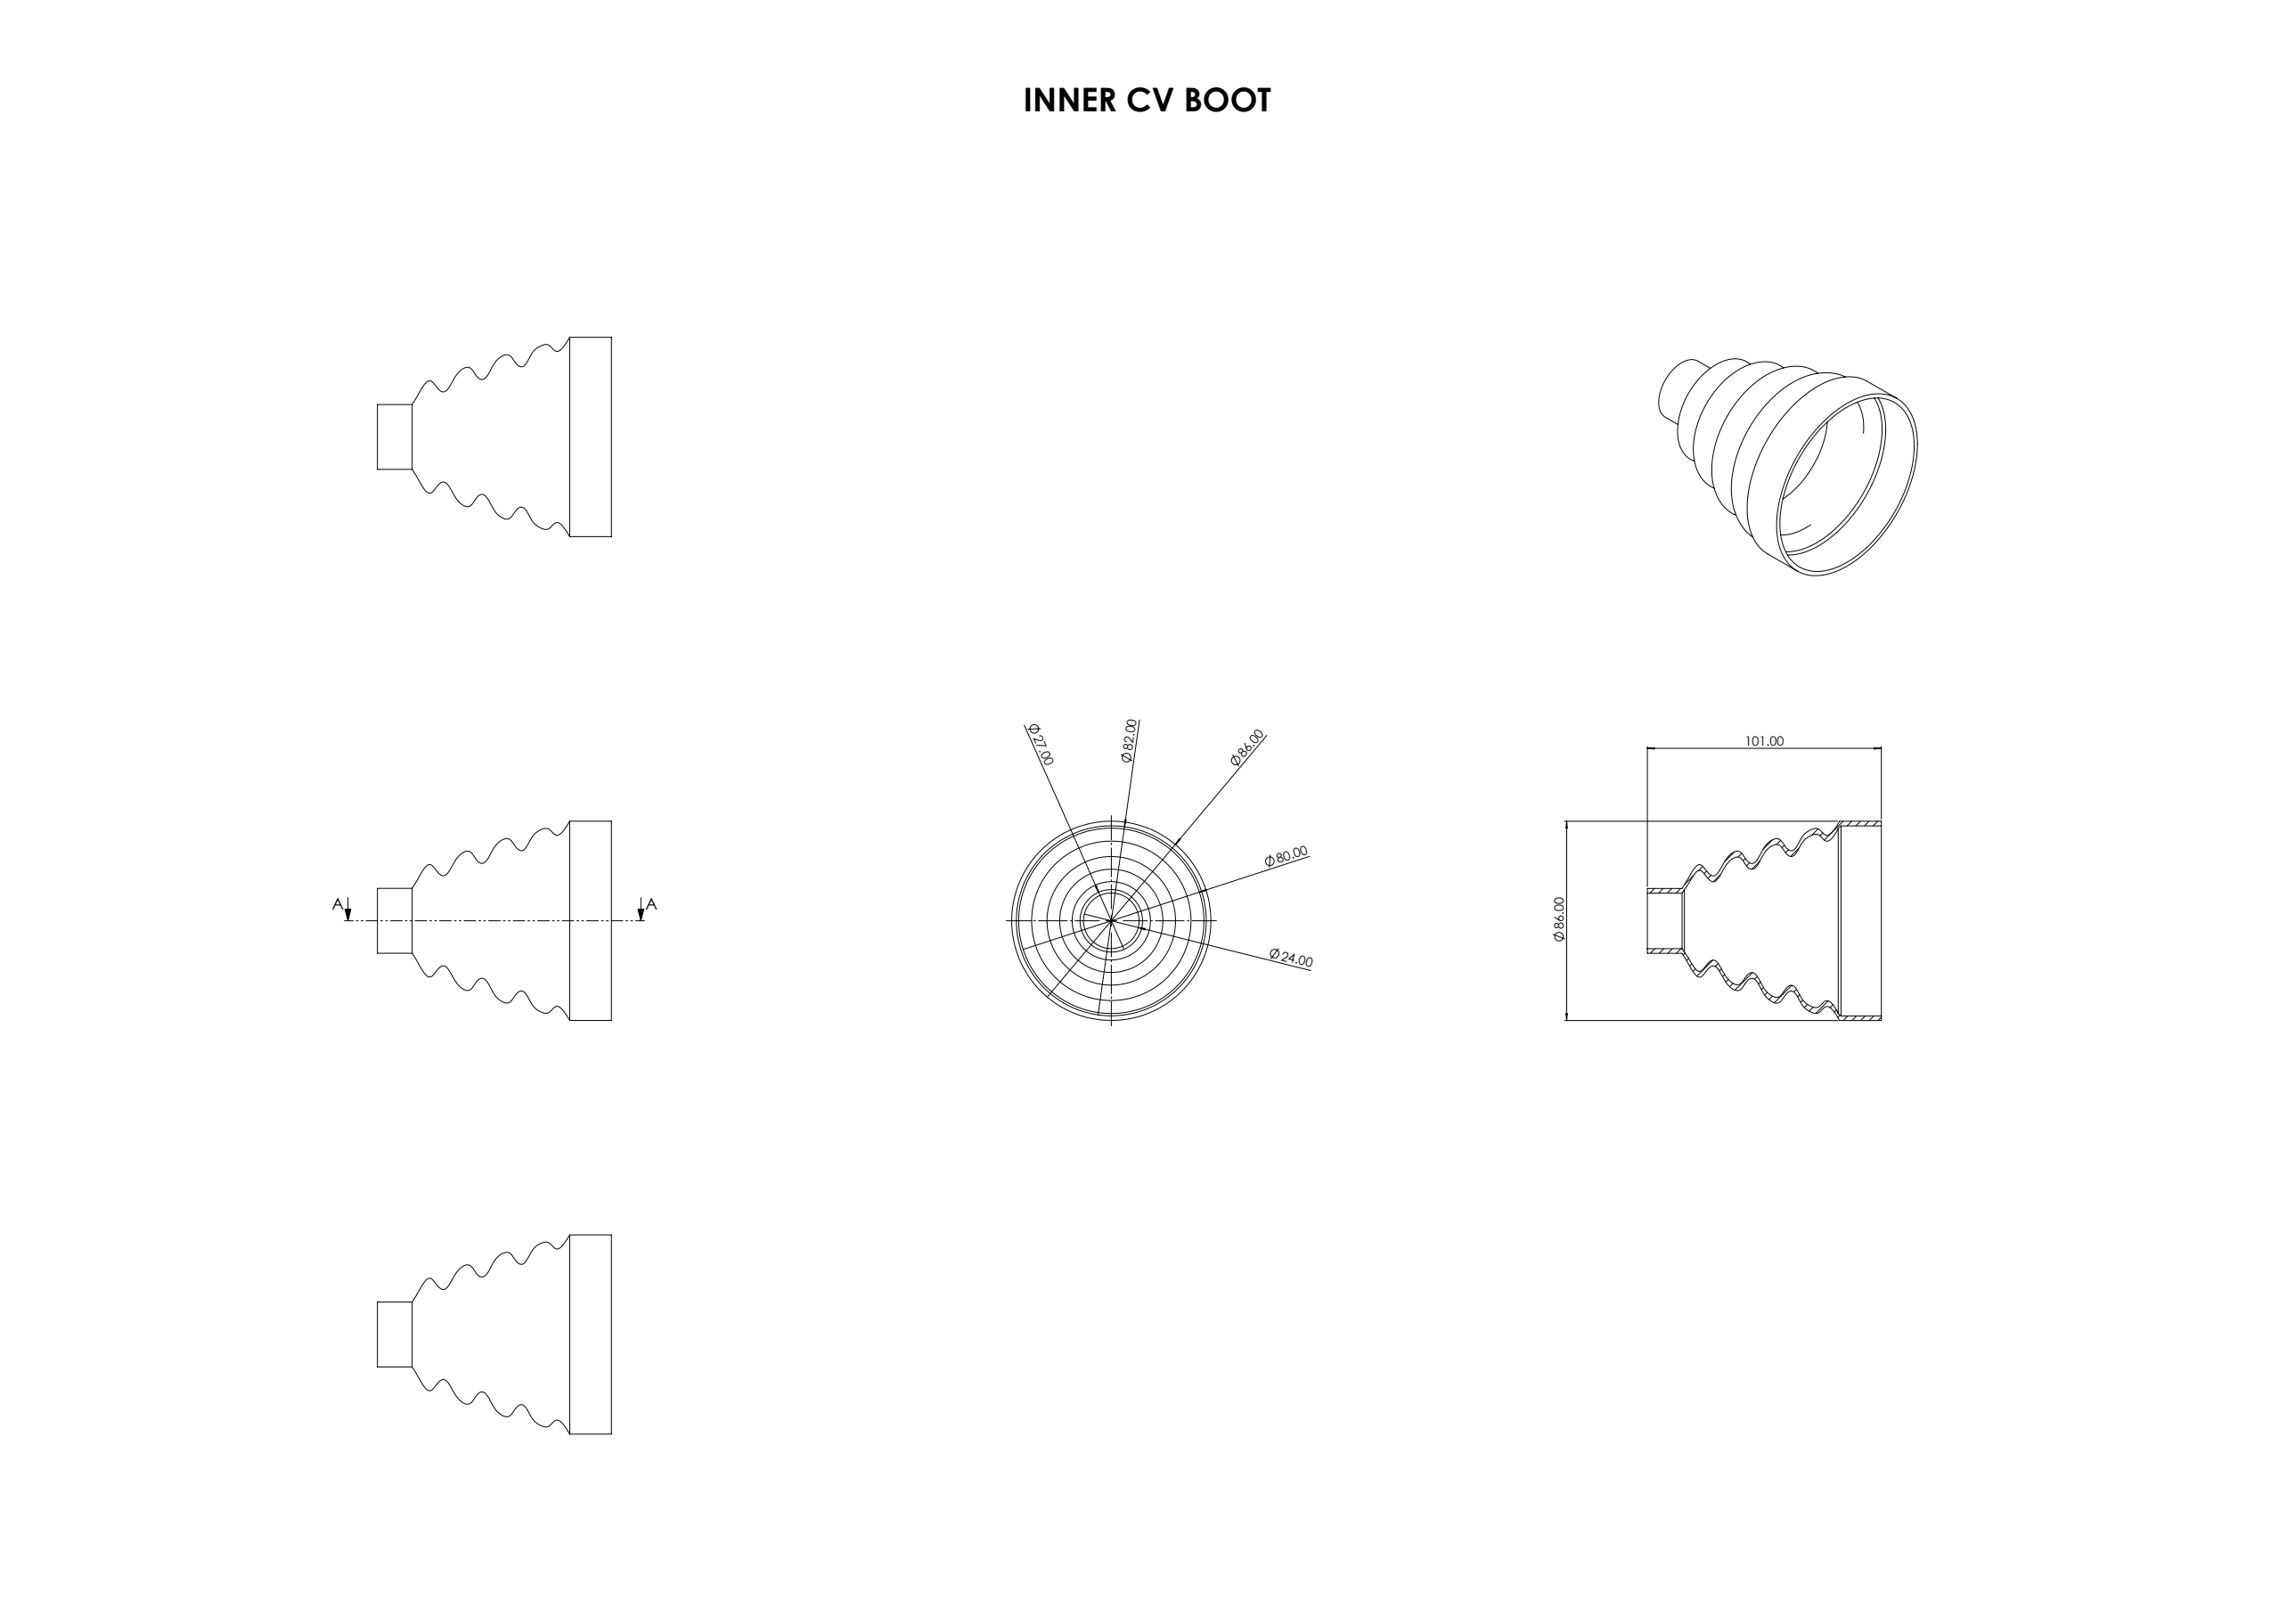
ISO-10303-21;
HEADER;
/* Generated by software containing ST-Developer
 * from STEP Tools, Inc. (www.steptools.com) 
 */

FILE_DESCRIPTION(
/* description */ (''),
/* implementation_level */ '2;1');

FILE_NAME(
/* name */ '11_Inner_CV_Boot.step',
/* time_stamp */ '2026-10-11T12:57:03-07:00',
/* author */ (''),
/* organization */ (''),
/* preprocessor_version */ 'ST-DEVELOPER v20.2',
/* originating_system */ 'Autodesk Translation Framework v15.15.0.0',
/* authorisation */ '');

FILE_SCHEMA (('AUTOMOTIVE_DESIGN { 1 0 10303 214 3 1 1 }'));
ENDSEC;

DATA;
#10=MECHANICAL_DESIGN_GEOMETRIC_PRESENTATION_REPRESENTATION('',(#266),#90374);
#232=SHAPE_REPRESENTATION_RELATIONSHIP('SRR','None',#90451,#249);
#249=ADVANCED_BREP_SHAPE_REPRESENTATION('',(#283),#90367);
#266=STYLED_ITEM('',(#90701),#283);
#283=MANIFOLD_SOLID_BREP('Body1',#40355);
#741=CONICAL_SURFACE('',#44252,40.5,0.694738276196683);
#742=CONICAL_SURFACE('',#44257,12.75,0.982793723247323);
#1073=FACE_BOUND('',#6504,.T.);
#1074=FACE_BOUND('',#6509,.T.);
#1637=PLANE('',#44239);
#1638=PLANE('',#44248);
#1929=(
BOUNDED_CURVE()
B_SPLINE_CURVE(5,(#85669,#85670,#85671,#85672,#85673,#85674,#85675,#85676,
#85677,#85678,#85679,#85680,#85681,#85682,#85683,#85684,#85685,#85686,#85687,
#85688,#85689,#85690,#85691,#85692,#85693,#85694,#85695,#85696,#85697,#85698,
#85699,#85700,#85701,#85702,#85703,#85704,#85705,#85706,#85707,#85708,#85709,
#85710,#85711,#85712,#85713,#85714,#85715,#85716,#85717,#85718,#85719,#85720,
#85721,#85722,#85723,#85724,#85725,#85726,#85727,#85728,#85729,#85730,#85731,
#85732,#85733,#85734,#85735,#85736,#85737,#85738,#85739,#85740,#85741,#85742,
#85743,#85744,#85745,#85746,#85747,#85748,#85749,#85750,#85751,#85752,#85753,
#85754,#85755,#85756,#85757,#85758,#85759,#85760,#85761,#85762,#85763,#85764,
#85765,#85766,#85767,#85768,#85769,#85770,#85771,#85772,#85773,#85774,#85775,
#85776,#85777,#85778),.UNSPECIFIED.,.F.,.F.)
B_SPLINE_CURVE_WITH_KNOTS((6,1,1,1,1,1,1,1,1,1,1,1,1,1,1,1,1,1,1,1,1,1,
1,1,1,1,1,1,1,1,1,1,1,1,1,1,1,1,1,1,1,1,1,1,1,1,1,1,1,1,1,1,1,1,1,1,1,1,
1,1,1,1,1,1,1,1,1,1,1,1,1,1,1,1,1,1,1,1,1,1,1,1,1,1,1,1,1,1,1,1,1,1,1,1,
1,1,1,1,1,1,1,1,1,1,1,6),(0.,0.00952380952380952,0.019047619047619,0.0285714285714286,
0.0380952380952381,0.0476190476190476,0.0571428571428571,0.0666666666666667,
0.0761904761904762,0.0857142857142857,0.0952380952380952,0.104761904761905,
0.114285714285714,0.123809523809524,0.133333333333333,0.142857142857143,
0.152380952380952,0.161904761904762,0.171428571428571,0.180952380952381,
0.19047619047619,0.2,0.209523809523809,0.219047619047619,0.228571428571428,
0.238095238095238,0.247619047619048,0.257142857142857,0.266666666666667,
0.276190476190476,0.285714285714286,0.295238095238095,0.304761904761905,
0.314285714285714,0.323809523809524,0.333333333333333,0.342857142857143,
0.352380952380953,0.361904761904762,0.371428571428572,0.380952380952381,
0.390476190476191,0.4,0.40952380952381,0.419047619047619,0.428571428571429,
0.438095238095238,0.447619047619048,0.457142857142858,0.466666666666667,
0.476190476190477,0.485714285714286,0.495238095238096,0.504761904761905,
0.514285714285715,0.523809523809524,0.533333333333334,0.542857142857143,
0.552380952380953,0.561904761904762,0.571428571428572,0.580952380952381,
0.590476190476191,0.6,0.60952380952381,0.619047619047619,0.628571428571429,
0.638095238095238,0.647619047619048,0.657142857142857,0.666666666666667,
0.676190476190476,0.685714285714285,0.695238095238095,0.704761904761904,
0.714285714285714,0.723809523809523,0.733333333333333,0.742857142857142,
0.752380952380952,0.761904761904761,0.771428571428571,0.78095238095238,
0.79047619047619,0.799999999999999,0.809523809523809,0.819047619047618,
0.828571428571428,0.838095238095237,0.847619047619047,0.857142857142856,
0.866666666666666,0.876190476190475,0.885714285714285,0.895238095238094,
0.904761904761904,0.914285714285713,0.923809523809523,0.933333333333332,
0.942857142857142,0.952380952380951,0.961904761904761,0.97142857142857,
0.98095238095238,0.990476190476189,1.),.UNSPECIFIED.)
CURVE()
GEOMETRIC_REPRESENTATION_ITEM()
RATIONAL_B_SPLINE_CURVE((1.,1.,1.,1.,1.,1.,1.,1.,1.,1.,1.,1.,1.,1.,1.,1.,
1.,1.,1.,1.,1.,1.,1.,1.,1.,1.,1.,1.,1.,1.,1.,1.,1.,1.,1.,1.,1.,1.,1.,1.,
1.,1.,1.,1.,1.,1.,1.,1.,1.,1.,1.,1.,1.,1.,1.,1.,1.,1.,1.,1.,1.,1.,1.,1.,
1.,1.,1.,1.,1.,1.,1.,1.,1.,1.,1.,1.,1.,1.,1.,1.,1.,1.,1.,1.,1.,1.,1.,1.,
1.,1.,1.,1.,1.,1.,1.,1.,1.,1.,1.,1.,1.,1.,1.,1.,1.,1.,1.,1.,1.,1.))
REPRESENTATION_ITEM('')
);
#1930=(
BOUNDED_CURVE()
B_SPLINE_CURVE(5,(#86790,#86791,#86792,#86793,#86794,#86795,#86796,#86797,
#86798,#86799,#86800,#86801,#86802,#86803,#86804,#86805,#86806,#86807,#86808,
#86809,#86810,#86811,#86812,#86813,#86814,#86815,#86816,#86817,#86818,#86819,
#86820,#86821,#86822,#86823,#86824,#86825,#86826,#86827,#86828,#86829,#86830,
#86831,#86832,#86833,#86834,#86835,#86836,#86837,#86838,#86839,#86840,#86841,
#86842,#86843,#86844,#86845,#86846,#86847,#86848,#86849,#86850,#86851,#86852,
#86853,#86854,#86855,#86856,#86857,#86858,#86859,#86860,#86861,#86862,#86863,
#86864,#86865,#86866,#86867,#86868,#86869,#86870,#86871,#86872,#86873,#86874,
#86875,#86876,#86877,#86878,#86879,#86880,#86881,#86882,#86883,#86884,#86885,
#86886,#86887,#86888,#86889,#86890,#86891,#86892,#86893,#86894,#86895,#86896,
#86897,#86898,#86899),.UNSPECIFIED.,.F.,.F.)
B_SPLINE_CURVE_WITH_KNOTS((6,1,1,1,1,1,1,1,1,1,1,1,1,1,1,1,1,1,1,1,1,1,
1,1,1,1,1,1,1,1,1,1,1,1,1,1,1,1,1,1,1,1,1,1,1,1,1,1,1,1,1,1,1,1,1,1,1,1,
1,1,1,1,1,1,1,1,1,1,1,1,1,1,1,1,1,1,1,1,1,1,1,1,1,1,1,1,1,1,1,1,1,1,1,1,
1,1,1,1,1,1,1,1,1,1,1,6),(0.,0.00952380952380952,0.019047619047619,0.0285714285714286,
0.0380952380952381,0.0476190476190476,0.0571428571428571,0.0666666666666667,
0.0761904761904762,0.0857142857142857,0.0952380952380952,0.104761904761905,
0.114285714285714,0.123809523809524,0.133333333333333,0.142857142857143,
0.152380952380952,0.161904761904762,0.171428571428571,0.180952380952381,
0.19047619047619,0.2,0.209523809523809,0.219047619047619,0.228571428571428,
0.238095238095238,0.247619047619048,0.257142857142857,0.266666666666667,
0.276190476190476,0.285714285714286,0.295238095238095,0.304761904761905,
0.314285714285714,0.323809523809524,0.333333333333333,0.342857142857143,
0.352380952380953,0.361904761904762,0.371428571428572,0.380952380952381,
0.390476190476191,0.4,0.40952380952381,0.419047619047619,0.428571428571429,
0.438095238095238,0.447619047619048,0.457142857142858,0.466666666666667,
0.476190476190477,0.485714285714286,0.495238095238096,0.504761904761905,
0.514285714285715,0.523809523809524,0.533333333333334,0.542857142857143,
0.552380952380953,0.561904761904762,0.571428571428572,0.580952380952381,
0.590476190476191,0.6,0.60952380952381,0.619047619047619,0.628571428571429,
0.638095238095238,0.647619047619048,0.657142857142857,0.666666666666667,
0.676190476190476,0.685714285714285,0.695238095238095,0.704761904761904,
0.714285714285714,0.723809523809523,0.733333333333333,0.742857142857142,
0.752380952380952,0.761904761904761,0.771428571428571,0.78095238095238,
0.79047619047619,0.799999999999999,0.809523809523809,0.819047619047618,
0.828571428571428,0.838095238095237,0.847619047619047,0.857142857142856,
0.866666666666666,0.876190476190475,0.885714285714285,0.895238095238094,
0.904761904761904,0.914285714285713,0.923809523809523,0.933333333333332,
0.942857142857142,0.952380952380951,0.961904761904761,0.97142857142857,
0.98095238095238,0.990476190476189,1.),.UNSPECIFIED.)
CURVE()
GEOMETRIC_REPRESENTATION_ITEM()
RATIONAL_B_SPLINE_CURVE((1.,1.,1.,1.,1.,1.,1.,1.,1.,1.,1.,1.,1.,1.,1.,1.,
1.,1.,1.,1.,1.,1.,1.,1.,1.,1.,1.,1.,1.,1.,1.,1.,1.,1.,1.,1.,1.,1.,1.,1.,
1.,1.,1.,1.,1.,1.,1.,1.,1.,1.,1.,1.,1.,1.,1.,1.,1.,1.,1.,1.,1.,1.,1.,1.,
1.,1.,1.,1.,1.,1.,1.,1.,1.,1.,1.,1.,1.,1.,1.,1.,1.,1.,1.,1.,1.,1.,1.,1.,
1.,1.,1.,1.,1.,1.,1.,1.,1.,1.,1.,1.,1.,1.,1.,1.,1.,1.,1.,1.,1.,1.))
REPRESENTATION_ITEM('')
);
#1936=(
BOUNDED_SURFACE()
B_SPLINE_SURFACE(5,2,((#84678,#84679,#84680,#84681,#84682,#84683,#84684,
#84685,#84686),(#84687,#84688,#84689,#84690,#84691,#84692,#84693,#84694,
#84695),(#84696,#84697,#84698,#84699,#84700,#84701,#84702,#84703,#84704),
(#84705,#84706,#84707,#84708,#84709,#84710,#84711,#84712,#84713),(#84714,
#84715,#84716,#84717,#84718,#84719,#84720,#84721,#84722),(#84723,#84724,
#84725,#84726,#84727,#84728,#84729,#84730,#84731),(#84732,#84733,#84734,
#84735,#84736,#84737,#84738,#84739,#84740),(#84741,#84742,#84743,#84744,
#84745,#84746,#84747,#84748,#84749),(#84750,#84751,#84752,#84753,#84754,
#84755,#84756,#84757,#84758),(#84759,#84760,#84761,#84762,#84763,#84764,
#84765,#84766,#84767),(#84768,#84769,#84770,#84771,#84772,#84773,#84774,
#84775,#84776),(#84777,#84778,#84779,#84780,#84781,#84782,#84783,#84784,
#84785),(#84786,#84787,#84788,#84789,#84790,#84791,#84792,#84793,#84794),
(#84795,#84796,#84797,#84798,#84799,#84800,#84801,#84802,#84803),(#84804,
#84805,#84806,#84807,#84808,#84809,#84810,#84811,#84812),(#84813,#84814,
#84815,#84816,#84817,#84818,#84819,#84820,#84821),(#84822,#84823,#84824,
#84825,#84826,#84827,#84828,#84829,#84830),(#84831,#84832,#84833,#84834,
#84835,#84836,#84837,#84838,#84839),(#84840,#84841,#84842,#84843,#84844,
#84845,#84846,#84847,#84848),(#84849,#84850,#84851,#84852,#84853,#84854,
#84855,#84856,#84857),(#84858,#84859,#84860,#84861,#84862,#84863,#84864,
#84865,#84866),(#84867,#84868,#84869,#84870,#84871,#84872,#84873,#84874,
#84875),(#84876,#84877,#84878,#84879,#84880,#84881,#84882,#84883,#84884),
(#84885,#84886,#84887,#84888,#84889,#84890,#84891,#84892,#84893),(#84894,
#84895,#84896,#84897,#84898,#84899,#84900,#84901,#84902),(#84903,#84904,
#84905,#84906,#84907,#84908,#84909,#84910,#84911),(#84912,#84913,#84914,
#84915,#84916,#84917,#84918,#84919,#84920),(#84921,#84922,#84923,#84924,
#84925,#84926,#84927,#84928,#84929),(#84930,#84931,#84932,#84933,#84934,
#84935,#84936,#84937,#84938),(#84939,#84940,#84941,#84942,#84943,#84944,
#84945,#84946,#84947),(#84948,#84949,#84950,#84951,#84952,#84953,#84954,
#84955,#84956),(#84957,#84958,#84959,#84960,#84961,#84962,#84963,#84964,
#84965),(#84966,#84967,#84968,#84969,#84970,#84971,#84972,#84973,#84974),
(#84975,#84976,#84977,#84978,#84979,#84980,#84981,#84982,#84983),(#84984,
#84985,#84986,#84987,#84988,#84989,#84990,#84991,#84992),(#84993,#84994,
#84995,#84996,#84997,#84998,#84999,#85000,#85001),(#85002,#85003,#85004,
#85005,#85006,#85007,#85008,#85009,#85010),(#85011,#85012,#85013,#85014,
#85015,#85016,#85017,#85018,#85019),(#85020,#85021,#85022,#85023,#85024,
#85025,#85026,#85027,#85028),(#85029,#85030,#85031,#85032,#85033,#85034,
#85035,#85036,#85037),(#85038,#85039,#85040,#85041,#85042,#85043,#85044,
#85045,#85046),(#85047,#85048,#85049,#85050,#85051,#85052,#85053,#85054,
#85055),(#85056,#85057,#85058,#85059,#85060,#85061,#85062,#85063,#85064),
(#85065,#85066,#85067,#85068,#85069,#85070,#85071,#85072,#85073),(#85074,
#85075,#85076,#85077,#85078,#85079,#85080,#85081,#85082),(#85083,#85084,
#85085,#85086,#85087,#85088,#85089,#85090,#85091),(#85092,#85093,#85094,
#85095,#85096,#85097,#85098,#85099,#85100),(#85101,#85102,#85103,#85104,
#85105,#85106,#85107,#85108,#85109),(#85110,#85111,#85112,#85113,#85114,
#85115,#85116,#85117,#85118),(#85119,#85120,#85121,#85122,#85123,#85124,
#85125,#85126,#85127),(#85128,#85129,#85130,#85131,#85132,#85133,#85134,
#85135,#85136),(#85137,#85138,#85139,#85140,#85141,#85142,#85143,#85144,
#85145),(#85146,#85147,#85148,#85149,#85150,#85151,#85152,#85153,#85154),
(#85155,#85156,#85157,#85158,#85159,#85160,#85161,#85162,#85163),(#85164,
#85165,#85166,#85167,#85168,#85169,#85170,#85171,#85172),(#85173,#85174,
#85175,#85176,#85177,#85178,#85179,#85180,#85181),(#85182,#85183,#85184,
#85185,#85186,#85187,#85188,#85189,#85190),(#85191,#85192,#85193,#85194,
#85195,#85196,#85197,#85198,#85199),(#85200,#85201,#85202,#85203,#85204,
#85205,#85206,#85207,#85208),(#85209,#85210,#85211,#85212,#85213,#85214,
#85215,#85216,#85217),(#85218,#85219,#85220,#85221,#85222,#85223,#85224,
#85225,#85226),(#85227,#85228,#85229,#85230,#85231,#85232,#85233,#85234,
#85235),(#85236,#85237,#85238,#85239,#85240,#85241,#85242,#85243,#85244),
(#85245,#85246,#85247,#85248,#85249,#85250,#85251,#85252,#85253),(#85254,
#85255,#85256,#85257,#85258,#85259,#85260,#85261,#85262),(#85263,#85264,
#85265,#85266,#85267,#85268,#85269,#85270,#85271),(#85272,#85273,#85274,
#85275,#85276,#85277,#85278,#85279,#85280),(#85281,#85282,#85283,#85284,
#85285,#85286,#85287,#85288,#85289),(#85290,#85291,#85292,#85293,#85294,
#85295,#85296,#85297,#85298),(#85299,#85300,#85301,#85302,#85303,#85304,
#85305,#85306,#85307),(#85308,#85309,#85310,#85311,#85312,#85313,#85314,
#85315,#85316),(#85317,#85318,#85319,#85320,#85321,#85322,#85323,#85324,
#85325),(#85326,#85327,#85328,#85329,#85330,#85331,#85332,#85333,#85334),
(#85335,#85336,#85337,#85338,#85339,#85340,#85341,#85342,#85343),(#85344,
#85345,#85346,#85347,#85348,#85349,#85350,#85351,#85352),(#85353,#85354,
#85355,#85356,#85357,#85358,#85359,#85360,#85361),(#85362,#85363,#85364,
#85365,#85366,#85367,#85368,#85369,#85370),(#85371,#85372,#85373,#85374,
#85375,#85376,#85377,#85378,#85379),(#85380,#85381,#85382,#85383,#85384,
#85385,#85386,#85387,#85388),(#85389,#85390,#85391,#85392,#85393,#85394,
#85395,#85396,#85397),(#85398,#85399,#85400,#85401,#85402,#85403,#85404,
#85405,#85406),(#85407,#85408,#85409,#85410,#85411,#85412,#85413,#85414,
#85415),(#85416,#85417,#85418,#85419,#85420,#85421,#85422,#85423,#85424),
(#85425,#85426,#85427,#85428,#85429,#85430,#85431,#85432,#85433),(#85434,
#85435,#85436,#85437,#85438,#85439,#85440,#85441,#85442),(#85443,#85444,
#85445,#85446,#85447,#85448,#85449,#85450,#85451),(#85452,#85453,#85454,
#85455,#85456,#85457,#85458,#85459,#85460),(#85461,#85462,#85463,#85464,
#85465,#85466,#85467,#85468,#85469),(#85470,#85471,#85472,#85473,#85474,
#85475,#85476,#85477,#85478),(#85479,#85480,#85481,#85482,#85483,#85484,
#85485,#85486,#85487),(#85488,#85489,#85490,#85491,#85492,#85493,#85494,
#85495,#85496),(#85497,#85498,#85499,#85500,#85501,#85502,#85503,#85504,
#85505),(#85506,#85507,#85508,#85509,#85510,#85511,#85512,#85513,#85514),
(#85515,#85516,#85517,#85518,#85519,#85520,#85521,#85522,#85523),(#85524,
#85525,#85526,#85527,#85528,#85529,#85530,#85531,#85532),(#85533,#85534,
#85535,#85536,#85537,#85538,#85539,#85540,#85541),(#85542,#85543,#85544,
#85545,#85546,#85547,#85548,#85549,#85550),(#85551,#85552,#85553,#85554,
#85555,#85556,#85557,#85558,#85559),(#85560,#85561,#85562,#85563,#85564,
#85565,#85566,#85567,#85568),(#85569,#85570,#85571,#85572,#85573,#85574,
#85575,#85576,#85577),(#85578,#85579,#85580,#85581,#85582,#85583,#85584,
#85585,#85586),(#85587,#85588,#85589,#85590,#85591,#85592,#85593,#85594,
#85595),(#85596,#85597,#85598,#85599,#85600,#85601,#85602,#85603,#85604),
(#85605,#85606,#85607,#85608,#85609,#85610,#85611,#85612,#85613),(#85614,
#85615,#85616,#85617,#85618,#85619,#85620,#85621,#85622),(#85623,#85624,
#85625,#85626,#85627,#85628,#85629,#85630,#85631),(#85632,#85633,#85634,
#85635,#85636,#85637,#85638,#85639,#85640),(#85641,#85642,#85643,#85644,
#85645,#85646,#85647,#85648,#85649),(#85650,#85651,#85652,#85653,#85654,
#85655,#85656,#85657,#85658),(#85659,#85660,#85661,#85662,#85663,#85664,
#85665,#85666,#85667)),.UNSPECIFIED.,.F.,.T.,.F.)
B_SPLINE_SURFACE_WITH_KNOTS((6,1,1,1,1,1,1,1,1,1,1,1,1,1,1,1,1,1,1,1,1,
1,1,1,1,1,1,1,1,1,1,1,1,1,1,1,1,1,1,1,1,1,1,1,1,1,1,1,1,1,1,1,1,1,1,1,1,
1,1,1,1,1,1,1,1,1,1,1,1,1,1,1,1,1,1,1,1,1,1,1,1,1,1,1,1,1,1,1,1,1,1,1,1,
1,1,1,1,1,1,1,1,1,1,1,1,6),(3,2,2,2,3),(-1.,-0.990476190476189,-0.98095238095238,
-0.97142857142857,-0.961904761904761,-0.952380952380951,-0.942857142857142,
-0.933333333333332,-0.923809523809523,-0.914285714285713,-0.904761904761904,
-0.895238095238094,-0.885714285714285,-0.876190476190475,-0.866666666666666,
-0.857142857142856,-0.847619047619047,-0.838095238095237,-0.828571428571428,
-0.819047619047618,-0.809523809523809,-0.799999999999999,-0.79047619047619,
-0.78095238095238,-0.771428571428571,-0.761904761904761,-0.752380952380952,
-0.742857142857142,-0.733333333333333,-0.723809523809523,-0.714285714285714,
-0.704761904761904,-0.695238095238095,-0.685714285714285,-0.676190476190476,
-0.666666666666667,-0.657142857142857,-0.647619047619048,-0.638095238095238,
-0.628571428571429,-0.619047619047619,-0.60952380952381,-0.6,-0.590476190476191,
-0.580952380952381,-0.571428571428572,-0.561904761904762,-0.552380952380953,
-0.542857142857143,-0.533333333333334,-0.523809523809524,-0.514285714285715,
-0.504761904761905,-0.495238095238096,-0.485714285714286,-0.476190476190477,
-0.466666666666667,-0.457142857142858,-0.447619047619048,-0.438095238095238,
-0.428571428571429,-0.419047619047619,-0.40952380952381,-0.4,-0.390476190476191,
-0.380952380952381,-0.371428571428572,-0.361904761904762,-0.352380952380953,
-0.342857142857143,-0.333333333333333,-0.323809523809524,-0.314285714285714,
-0.304761904761905,-0.295238095238095,-0.285714285714286,-0.276190476190476,
-0.266666666666667,-0.257142857142857,-0.247619047619048,-0.238095238095238,
-0.228571428571428,-0.219047619047619,-0.209523809523809,-0.2,-0.19047619047619,
-0.180952380952381,-0.171428571428571,-0.161904761904762,-0.152380952380952,
-0.142857142857143,-0.133333333333333,-0.123809523809524,-0.114285714285714,
-0.104761904761905,-0.0952380952380952,-0.0857142857142857,-0.0761904761904762,
-0.0666666666666667,-0.0571428571428571,-0.0476190476190476,-0.0380952380952381,
-0.0285714285714286,-0.019047619047619,-0.00952380952380952,0.),(0.,1.5707963267949,
3.14159265358979,4.71238898038469,6.28318530717959),.UNSPECIFIED.)
GEOMETRIC_REPRESENTATION_ITEM()
RATIONAL_B_SPLINE_SURFACE(((1.,0.707106781186548,1.,0.707106781186548,1.,
0.707106781186548,1.,0.707106781186548,1.),(1.,0.707106781186548,1.,0.707106781186548,
1.,0.707106781186548,1.,0.707106781186548,1.),(1.,0.707106781186548,1.,
0.707106781186548,1.,0.707106781186548,1.,0.707106781186548,1.),(1.,0.707106781186548,
1.,0.707106781186548,1.,0.707106781186548,1.,0.707106781186548,1.),(1.,
0.707106781186548,1.,0.707106781186548,1.,0.707106781186548,1.,0.707106781186548,
1.),(1.,0.707106781186548,1.,0.707106781186548,1.,0.707106781186548,1.,
0.707106781186548,1.),(1.,0.707106781186548,1.,0.707106781186548,1.,0.707106781186548,
1.,0.707106781186548,1.),(1.,0.707106781186548,1.,0.707106781186548,1.,
0.707106781186548,1.,0.707106781186548,1.),(1.,0.707106781186548,1.,0.707106781186548,
1.,0.707106781186548,1.,0.707106781186548,1.),(1.,0.707106781186548,1.,
0.707106781186548,1.,0.707106781186548,1.,0.707106781186548,1.),(1.,0.707106781186548,
1.,0.707106781186548,1.,0.707106781186548,1.,0.707106781186548,1.),(1.,
0.707106781186548,1.,0.707106781186548,1.,0.707106781186548,1.,0.707106781186548,
1.),(1.,0.707106781186548,1.,0.707106781186548,1.,0.707106781186548,1.,
0.707106781186548,1.),(1.,0.707106781186548,1.,0.707106781186548,1.,0.707106781186548,
1.,0.707106781186548,1.),(1.,0.707106781186548,1.,0.707106781186548,1.,
0.707106781186548,1.,0.707106781186548,1.),(1.,0.707106781186548,1.,0.707106781186548,
1.,0.707106781186548,1.,0.707106781186548,1.),(1.,0.707106781186548,1.,
0.707106781186548,1.,0.707106781186548,1.,0.707106781186548,1.),(1.,0.707106781186548,
1.,0.707106781186548,1.,0.707106781186548,1.,0.707106781186548,1.),(1.,
0.707106781186548,1.,0.707106781186548,1.,0.707106781186548,1.,0.707106781186548,
1.),(1.,0.707106781186548,1.,0.707106781186548,1.,0.707106781186548,1.,
0.707106781186548,1.),(1.,0.707106781186548,1.,0.707106781186548,1.,0.707106781186548,
1.,0.707106781186548,1.),(1.,0.707106781186548,1.,0.707106781186548,1.,
0.707106781186548,1.,0.707106781186548,1.),(1.,0.707106781186548,1.,0.707106781186548,
1.,0.707106781186548,1.,0.707106781186548,1.),(1.,0.707106781186548,1.,
0.707106781186548,1.,0.707106781186548,1.,0.707106781186548,1.),(1.,0.707106781186548,
1.,0.707106781186548,1.,0.707106781186548,1.,0.707106781186548,1.),(1.,
0.707106781186548,1.,0.707106781186548,1.,0.707106781186548,1.,0.707106781186548,
1.),(1.,0.707106781186548,1.,0.707106781186548,1.,0.707106781186548,1.,
0.707106781186548,1.),(1.,0.707106781186548,1.,0.707106781186548,1.,0.707106781186548,
1.,0.707106781186548,1.),(1.,0.707106781186548,1.,0.707106781186548,1.,
0.707106781186548,1.,0.707106781186548,1.),(1.,0.707106781186548,1.,0.707106781186548,
1.,0.707106781186548,1.,0.707106781186548,1.),(1.,0.707106781186548,1.,
0.707106781186548,1.,0.707106781186548,1.,0.707106781186548,1.),(1.,0.707106781186548,
1.,0.707106781186548,1.,0.707106781186548,1.,0.707106781186548,1.),(1.,
0.707106781186548,1.,0.707106781186548,1.,0.707106781186548,1.,0.707106781186548,
1.),(1.,0.707106781186548,1.,0.707106781186548,1.,0.707106781186548,1.,
0.707106781186548,1.),(1.,0.707106781186548,1.,0.707106781186548,1.,0.707106781186548,
1.,0.707106781186548,1.),(1.,0.707106781186548,1.,0.707106781186548,1.,
0.707106781186548,1.,0.707106781186548,1.),(1.,0.707106781186548,1.,0.707106781186548,
1.,0.707106781186548,1.,0.707106781186548,1.),(1.,0.707106781186548,1.,
0.707106781186548,1.,0.707106781186548,1.,0.707106781186548,1.),(1.,0.707106781186548,
1.,0.707106781186548,1.,0.707106781186548,1.,0.707106781186548,1.),(1.,
0.707106781186548,1.,0.707106781186548,1.,0.707106781186548,1.,0.707106781186548,
1.),(1.,0.707106781186548,1.,0.707106781186548,1.,0.707106781186548,1.,
0.707106781186548,1.),(1.,0.707106781186548,1.,0.707106781186548,1.,0.707106781186548,
1.,0.707106781186548,1.),(1.,0.707106781186548,1.,0.707106781186548,1.,
0.707106781186548,1.,0.707106781186548,1.),(1.,0.707106781186548,1.,0.707106781186548,
1.,0.707106781186548,1.,0.707106781186548,1.),(1.,0.707106781186548,1.,
0.707106781186548,1.,0.707106781186548,1.,0.707106781186548,1.),(1.,0.707106781186548,
1.,0.707106781186548,1.,0.707106781186548,1.,0.707106781186548,1.),(1.,
0.707106781186548,1.,0.707106781186548,1.,0.707106781186548,1.,0.707106781186548,
1.),(1.,0.707106781186548,1.,0.707106781186548,1.,0.707106781186548,1.,
0.707106781186548,1.),(1.,0.707106781186548,1.,0.707106781186548,1.,0.707106781186548,
1.,0.707106781186548,1.),(1.,0.707106781186548,1.,0.707106781186548,1.,
0.707106781186548,1.,0.707106781186548,1.),(1.,0.707106781186548,1.,0.707106781186548,
1.,0.707106781186548,1.,0.707106781186548,1.),(1.,0.707106781186548,1.,
0.707106781186548,1.,0.707106781186548,1.,0.707106781186548,1.),(1.,0.707106781186548,
1.,0.707106781186548,1.,0.707106781186548,1.,0.707106781186548,1.),(1.,
0.707106781186548,1.,0.707106781186548,1.,0.707106781186548,1.,0.707106781186548,
1.),(1.,0.707106781186548,1.,0.707106781186548,1.,0.707106781186548,1.,
0.707106781186548,1.),(1.,0.707106781186548,1.,0.707106781186548,1.,0.707106781186548,
1.,0.707106781186548,1.),(1.,0.707106781186548,1.,0.707106781186548,1.,
0.707106781186548,1.,0.707106781186548,1.),(1.,0.707106781186548,1.,0.707106781186548,
1.,0.707106781186548,1.,0.707106781186548,1.),(1.,0.707106781186548,1.,
0.707106781186548,1.,0.707106781186548,1.,0.707106781186548,1.),(1.,0.707106781186548,
1.,0.707106781186548,1.,0.707106781186548,1.,0.707106781186548,1.),(1.,
0.707106781186548,1.,0.707106781186548,1.,0.707106781186548,1.,0.707106781186548,
1.),(1.,0.707106781186548,1.,0.707106781186548,1.,0.707106781186548,1.,
0.707106781186548,1.),(1.,0.707106781186548,1.,0.707106781186548,1.,0.707106781186548,
1.,0.707106781186548,1.),(1.,0.707106781186548,1.,0.707106781186548,1.,
0.707106781186548,1.,0.707106781186548,1.),(1.,0.707106781186548,1.,0.707106781186548,
1.,0.707106781186548,1.,0.707106781186548,1.),(1.,0.707106781186548,1.,
0.707106781186548,1.,0.707106781186548,1.,0.707106781186548,1.),(1.,0.707106781186548,
1.,0.707106781186548,1.,0.707106781186548,1.,0.707106781186548,1.),(1.,
0.707106781186548,1.,0.707106781186548,1.,0.707106781186548,1.,0.707106781186548,
1.),(1.,0.707106781186548,1.,0.707106781186548,1.,0.707106781186548,1.,
0.707106781186548,1.),(1.,0.707106781186548,1.,0.707106781186548,1.,0.707106781186548,
1.,0.707106781186548,1.),(1.,0.707106781186548,1.,0.707106781186548,1.,
0.707106781186548,1.,0.707106781186548,1.),(1.,0.707106781186548,1.,0.707106781186548,
1.,0.707106781186548,1.,0.707106781186548,1.),(1.,0.707106781186548,1.,
0.707106781186548,1.,0.707106781186548,1.,0.707106781186548,1.),(1.,0.707106781186548,
1.,0.707106781186548,1.,0.707106781186548,1.,0.707106781186548,1.),(1.,
0.707106781186548,1.,0.707106781186548,1.,0.707106781186548,1.,0.707106781186548,
1.),(1.,0.707106781186548,1.,0.707106781186548,1.,0.707106781186548,1.,
0.707106781186548,1.),(1.,0.707106781186548,1.,0.707106781186548,1.,0.707106781186548,
1.,0.707106781186548,1.),(1.,0.707106781186548,1.,0.707106781186548,1.,
0.707106781186548,1.,0.707106781186548,1.),(1.,0.707106781186548,1.,0.707106781186548,
1.,0.707106781186548,1.,0.707106781186548,1.),(1.,0.707106781186548,1.,
0.707106781186548,1.,0.707106781186548,1.,0.707106781186548,1.),(1.,0.707106781186548,
1.,0.707106781186548,1.,0.707106781186548,1.,0.707106781186548,1.),(1.,
0.707106781186548,1.,0.707106781186548,1.,0.707106781186548,1.,0.707106781186548,
1.),(1.,0.707106781186548,1.,0.707106781186548,1.,0.707106781186548,1.,
0.707106781186548,1.),(1.,0.707106781186548,1.,0.707106781186548,1.,0.707106781186548,
1.,0.707106781186548,1.),(1.,0.707106781186548,1.,0.707106781186548,1.,
0.707106781186548,1.,0.707106781186548,1.),(1.,0.707106781186548,1.,0.707106781186548,
1.,0.707106781186548,1.,0.707106781186548,1.),(1.,0.707106781186548,1.,
0.707106781186548,1.,0.707106781186548,1.,0.707106781186548,1.),(1.,0.707106781186548,
1.,0.707106781186548,1.,0.707106781186548,1.,0.707106781186548,1.),(1.,
0.707106781186548,1.,0.707106781186548,1.,0.707106781186548,1.,0.707106781186548,
1.),(1.,0.707106781186548,1.,0.707106781186548,1.,0.707106781186548,1.,
0.707106781186548,1.),(1.,0.707106781186548,1.,0.707106781186548,1.,0.707106781186548,
1.,0.707106781186548,1.),(1.,0.707106781186548,1.,0.707106781186548,1.,
0.707106781186548,1.,0.707106781186548,1.),(1.,0.707106781186548,1.,0.707106781186548,
1.,0.707106781186548,1.,0.707106781186548,1.),(1.,0.707106781186548,1.,
0.707106781186548,1.,0.707106781186548,1.,0.707106781186548,1.),(1.,0.707106781186548,
1.,0.707106781186548,1.,0.707106781186548,1.,0.707106781186548,1.),(1.,
0.707106781186548,1.,0.707106781186548,1.,0.707106781186548,1.,0.707106781186548,
1.),(1.,0.707106781186548,1.,0.707106781186548,1.,0.707106781186548,1.,
0.707106781186548,1.),(1.,0.707106781186548,1.,0.707106781186548,1.,0.707106781186548,
1.,0.707106781186548,1.),(1.,0.707106781186548,1.,0.707106781186548,1.,
0.707106781186548,1.,0.707106781186548,1.),(1.,0.707106781186548,1.,0.707106781186548,
1.,0.707106781186548,1.,0.707106781186548,1.),(1.,0.707106781186548,1.,
0.707106781186548,1.,0.707106781186548,1.,0.707106781186548,1.),(1.,0.707106781186548,
1.,0.707106781186548,1.,0.707106781186548,1.,0.707106781186548,1.),(1.,
0.707106781186548,1.,0.707106781186548,1.,0.707106781186548,1.,0.707106781186548,
1.),(1.,0.707106781186548,1.,0.707106781186548,1.,0.707106781186548,1.,
0.707106781186548,1.),(1.,0.707106781186548,1.,0.707106781186548,1.,0.707106781186548,
1.,0.707106781186548,1.),(1.,0.707106781186548,1.,0.707106781186548,1.,
0.707106781186548,1.,0.707106781186548,1.),(1.,0.707106781186548,1.,0.707106781186548,
1.,0.707106781186548,1.,0.707106781186548,1.),(1.,0.707106781186548,1.,
0.707106781186548,1.,0.707106781186548,1.,0.707106781186548,1.),(1.,0.707106781186548,
1.,0.707106781186548,1.,0.707106781186548,1.,0.707106781186548,1.),(1.,
0.707106781186548,1.,0.707106781186548,1.,0.707106781186548,1.,0.707106781186548,
1.)))
REPRESENTATION_ITEM('')
SURFACE()
);
#1937=(
BOUNDED_SURFACE()
B_SPLINE_SURFACE(5,2,((#85799,#85800,#85801,#85802,#85803,#85804,#85805,
#85806,#85807),(#85808,#85809,#85810,#85811,#85812,#85813,#85814,#85815,
#85816),(#85817,#85818,#85819,#85820,#85821,#85822,#85823,#85824,#85825),
(#85826,#85827,#85828,#85829,#85830,#85831,#85832,#85833,#85834),(#85835,
#85836,#85837,#85838,#85839,#85840,#85841,#85842,#85843),(#85844,#85845,
#85846,#85847,#85848,#85849,#85850,#85851,#85852),(#85853,#85854,#85855,
#85856,#85857,#85858,#85859,#85860,#85861),(#85862,#85863,#85864,#85865,
#85866,#85867,#85868,#85869,#85870),(#85871,#85872,#85873,#85874,#85875,
#85876,#85877,#85878,#85879),(#85880,#85881,#85882,#85883,#85884,#85885,
#85886,#85887,#85888),(#85889,#85890,#85891,#85892,#85893,#85894,#85895,
#85896,#85897),(#85898,#85899,#85900,#85901,#85902,#85903,#85904,#85905,
#85906),(#85907,#85908,#85909,#85910,#85911,#85912,#85913,#85914,#85915),
(#85916,#85917,#85918,#85919,#85920,#85921,#85922,#85923,#85924),(#85925,
#85926,#85927,#85928,#85929,#85930,#85931,#85932,#85933),(#85934,#85935,
#85936,#85937,#85938,#85939,#85940,#85941,#85942),(#85943,#85944,#85945,
#85946,#85947,#85948,#85949,#85950,#85951),(#85952,#85953,#85954,#85955,
#85956,#85957,#85958,#85959,#85960),(#85961,#85962,#85963,#85964,#85965,
#85966,#85967,#85968,#85969),(#85970,#85971,#85972,#85973,#85974,#85975,
#85976,#85977,#85978),(#85979,#85980,#85981,#85982,#85983,#85984,#85985,
#85986,#85987),(#85988,#85989,#85990,#85991,#85992,#85993,#85994,#85995,
#85996),(#85997,#85998,#85999,#86000,#86001,#86002,#86003,#86004,#86005),
(#86006,#86007,#86008,#86009,#86010,#86011,#86012,#86013,#86014),(#86015,
#86016,#86017,#86018,#86019,#86020,#86021,#86022,#86023),(#86024,#86025,
#86026,#86027,#86028,#86029,#86030,#86031,#86032),(#86033,#86034,#86035,
#86036,#86037,#86038,#86039,#86040,#86041),(#86042,#86043,#86044,#86045,
#86046,#86047,#86048,#86049,#86050),(#86051,#86052,#86053,#86054,#86055,
#86056,#86057,#86058,#86059),(#86060,#86061,#86062,#86063,#86064,#86065,
#86066,#86067,#86068),(#86069,#86070,#86071,#86072,#86073,#86074,#86075,
#86076,#86077),(#86078,#86079,#86080,#86081,#86082,#86083,#86084,#86085,
#86086),(#86087,#86088,#86089,#86090,#86091,#86092,#86093,#86094,#86095),
(#86096,#86097,#86098,#86099,#86100,#86101,#86102,#86103,#86104),(#86105,
#86106,#86107,#86108,#86109,#86110,#86111,#86112,#86113),(#86114,#86115,
#86116,#86117,#86118,#86119,#86120,#86121,#86122),(#86123,#86124,#86125,
#86126,#86127,#86128,#86129,#86130,#86131),(#86132,#86133,#86134,#86135,
#86136,#86137,#86138,#86139,#86140),(#86141,#86142,#86143,#86144,#86145,
#86146,#86147,#86148,#86149),(#86150,#86151,#86152,#86153,#86154,#86155,
#86156,#86157,#86158),(#86159,#86160,#86161,#86162,#86163,#86164,#86165,
#86166,#86167),(#86168,#86169,#86170,#86171,#86172,#86173,#86174,#86175,
#86176),(#86177,#86178,#86179,#86180,#86181,#86182,#86183,#86184,#86185),
(#86186,#86187,#86188,#86189,#86190,#86191,#86192,#86193,#86194),(#86195,
#86196,#86197,#86198,#86199,#86200,#86201,#86202,#86203),(#86204,#86205,
#86206,#86207,#86208,#86209,#86210,#86211,#86212),(#86213,#86214,#86215,
#86216,#86217,#86218,#86219,#86220,#86221),(#86222,#86223,#86224,#86225,
#86226,#86227,#86228,#86229,#86230),(#86231,#86232,#86233,#86234,#86235,
#86236,#86237,#86238,#86239),(#86240,#86241,#86242,#86243,#86244,#86245,
#86246,#86247,#86248),(#86249,#86250,#86251,#86252,#86253,#86254,#86255,
#86256,#86257),(#86258,#86259,#86260,#86261,#86262,#86263,#86264,#86265,
#86266),(#86267,#86268,#86269,#86270,#86271,#86272,#86273,#86274,#86275),
(#86276,#86277,#86278,#86279,#86280,#86281,#86282,#86283,#86284),(#86285,
#86286,#86287,#86288,#86289,#86290,#86291,#86292,#86293),(#86294,#86295,
#86296,#86297,#86298,#86299,#86300,#86301,#86302),(#86303,#86304,#86305,
#86306,#86307,#86308,#86309,#86310,#86311),(#86312,#86313,#86314,#86315,
#86316,#86317,#86318,#86319,#86320),(#86321,#86322,#86323,#86324,#86325,
#86326,#86327,#86328,#86329),(#86330,#86331,#86332,#86333,#86334,#86335,
#86336,#86337,#86338),(#86339,#86340,#86341,#86342,#86343,#86344,#86345,
#86346,#86347),(#86348,#86349,#86350,#86351,#86352,#86353,#86354,#86355,
#86356),(#86357,#86358,#86359,#86360,#86361,#86362,#86363,#86364,#86365),
(#86366,#86367,#86368,#86369,#86370,#86371,#86372,#86373,#86374),(#86375,
#86376,#86377,#86378,#86379,#86380,#86381,#86382,#86383),(#86384,#86385,
#86386,#86387,#86388,#86389,#86390,#86391,#86392),(#86393,#86394,#86395,
#86396,#86397,#86398,#86399,#86400,#86401),(#86402,#86403,#86404,#86405,
#86406,#86407,#86408,#86409,#86410),(#86411,#86412,#86413,#86414,#86415,
#86416,#86417,#86418,#86419),(#86420,#86421,#86422,#86423,#86424,#86425,
#86426,#86427,#86428),(#86429,#86430,#86431,#86432,#86433,#86434,#86435,
#86436,#86437),(#86438,#86439,#86440,#86441,#86442,#86443,#86444,#86445,
#86446),(#86447,#86448,#86449,#86450,#86451,#86452,#86453,#86454,#86455),
(#86456,#86457,#86458,#86459,#86460,#86461,#86462,#86463,#86464),(#86465,
#86466,#86467,#86468,#86469,#86470,#86471,#86472,#86473),(#86474,#86475,
#86476,#86477,#86478,#86479,#86480,#86481,#86482),(#86483,#86484,#86485,
#86486,#86487,#86488,#86489,#86490,#86491),(#86492,#86493,#86494,#86495,
#86496,#86497,#86498,#86499,#86500),(#86501,#86502,#86503,#86504,#86505,
#86506,#86507,#86508,#86509),(#86510,#86511,#86512,#86513,#86514,#86515,
#86516,#86517,#86518),(#86519,#86520,#86521,#86522,#86523,#86524,#86525,
#86526,#86527),(#86528,#86529,#86530,#86531,#86532,#86533,#86534,#86535,
#86536),(#86537,#86538,#86539,#86540,#86541,#86542,#86543,#86544,#86545),
(#86546,#86547,#86548,#86549,#86550,#86551,#86552,#86553,#86554),(#86555,
#86556,#86557,#86558,#86559,#86560,#86561,#86562,#86563),(#86564,#86565,
#86566,#86567,#86568,#86569,#86570,#86571,#86572),(#86573,#86574,#86575,
#86576,#86577,#86578,#86579,#86580,#86581),(#86582,#86583,#86584,#86585,
#86586,#86587,#86588,#86589,#86590),(#86591,#86592,#86593,#86594,#86595,
#86596,#86597,#86598,#86599),(#86600,#86601,#86602,#86603,#86604,#86605,
#86606,#86607,#86608),(#86609,#86610,#86611,#86612,#86613,#86614,#86615,
#86616,#86617),(#86618,#86619,#86620,#86621,#86622,#86623,#86624,#86625,
#86626),(#86627,#86628,#86629,#86630,#86631,#86632,#86633,#86634,#86635),
(#86636,#86637,#86638,#86639,#86640,#86641,#86642,#86643,#86644),(#86645,
#86646,#86647,#86648,#86649,#86650,#86651,#86652,#86653),(#86654,#86655,
#86656,#86657,#86658,#86659,#86660,#86661,#86662),(#86663,#86664,#86665,
#86666,#86667,#86668,#86669,#86670,#86671),(#86672,#86673,#86674,#86675,
#86676,#86677,#86678,#86679,#86680),(#86681,#86682,#86683,#86684,#86685,
#86686,#86687,#86688,#86689),(#86690,#86691,#86692,#86693,#86694,#86695,
#86696,#86697,#86698),(#86699,#86700,#86701,#86702,#86703,#86704,#86705,
#86706,#86707),(#86708,#86709,#86710,#86711,#86712,#86713,#86714,#86715,
#86716),(#86717,#86718,#86719,#86720,#86721,#86722,#86723,#86724,#86725),
(#86726,#86727,#86728,#86729,#86730,#86731,#86732,#86733,#86734),(#86735,
#86736,#86737,#86738,#86739,#86740,#86741,#86742,#86743),(#86744,#86745,
#86746,#86747,#86748,#86749,#86750,#86751,#86752),(#86753,#86754,#86755,
#86756,#86757,#86758,#86759,#86760,#86761),(#86762,#86763,#86764,#86765,
#86766,#86767,#86768,#86769,#86770),(#86771,#86772,#86773,#86774,#86775,
#86776,#86777,#86778,#86779),(#86780,#86781,#86782,#86783,#86784,#86785,
#86786,#86787,#86788)),.UNSPECIFIED.,.F.,.T.,.F.)
B_SPLINE_SURFACE_WITH_KNOTS((6,1,1,1,1,1,1,1,1,1,1,1,1,1,1,1,1,1,1,1,1,
1,1,1,1,1,1,1,1,1,1,1,1,1,1,1,1,1,1,1,1,1,1,1,1,1,1,1,1,1,1,1,1,1,1,1,1,
1,1,1,1,1,1,1,1,1,1,1,1,1,1,1,1,1,1,1,1,1,1,1,1,1,1,1,1,1,1,1,1,1,1,1,1,
1,1,1,1,1,1,1,1,1,1,1,1,6),(3,2,2,2,3),(-1.,-0.990476190476189,-0.98095238095238,
-0.97142857142857,-0.961904761904761,-0.952380952380951,-0.942857142857142,
-0.933333333333332,-0.923809523809523,-0.914285714285713,-0.904761904761904,
-0.895238095238094,-0.885714285714285,-0.876190476190475,-0.866666666666666,
-0.857142857142856,-0.847619047619047,-0.838095238095237,-0.828571428571428,
-0.819047619047618,-0.809523809523809,-0.799999999999999,-0.79047619047619,
-0.78095238095238,-0.771428571428571,-0.761904761904761,-0.752380952380952,
-0.742857142857142,-0.733333333333333,-0.723809523809523,-0.714285714285714,
-0.704761904761904,-0.695238095238095,-0.685714285714285,-0.676190476190476,
-0.666666666666667,-0.657142857142857,-0.647619047619048,-0.638095238095238,
-0.628571428571429,-0.619047619047619,-0.60952380952381,-0.6,-0.590476190476191,
-0.580952380952381,-0.571428571428572,-0.561904761904762,-0.552380952380953,
-0.542857142857143,-0.533333333333334,-0.523809523809524,-0.514285714285715,
-0.504761904761905,-0.495238095238096,-0.485714285714286,-0.476190476190477,
-0.466666666666667,-0.457142857142858,-0.447619047619048,-0.438095238095238,
-0.428571428571429,-0.419047619047619,-0.40952380952381,-0.4,-0.390476190476191,
-0.380952380952381,-0.371428571428572,-0.361904761904762,-0.352380952380953,
-0.342857142857143,-0.333333333333333,-0.323809523809524,-0.314285714285714,
-0.304761904761905,-0.295238095238095,-0.285714285714286,-0.276190476190476,
-0.266666666666667,-0.257142857142857,-0.247619047619048,-0.238095238095238,
-0.228571428571428,-0.219047619047619,-0.209523809523809,-0.2,-0.19047619047619,
-0.180952380952381,-0.171428571428571,-0.161904761904762,-0.152380952380952,
-0.142857142857143,-0.133333333333333,-0.123809523809524,-0.114285714285714,
-0.104761904761905,-0.0952380952380952,-0.0857142857142857,-0.0761904761904762,
-0.0666666666666667,-0.0571428571428571,-0.0476190476190476,-0.0380952380952381,
-0.0285714285714286,-0.019047619047619,-0.00952380952380952,0.),(0.,1.5707963267949,
3.14159265358979,4.71238898038469,6.28318530717959),.UNSPECIFIED.)
GEOMETRIC_REPRESENTATION_ITEM()
RATIONAL_B_SPLINE_SURFACE(((1.,0.707106781186548,1.,0.707106781186548,1.,
0.707106781186548,1.,0.707106781186548,1.),(1.,0.707106781186548,1.,0.707106781186548,
1.,0.707106781186548,1.,0.707106781186548,1.),(1.,0.707106781186548,1.,
0.707106781186548,1.,0.707106781186548,1.,0.707106781186548,1.),(1.,0.707106781186548,
1.,0.707106781186548,1.,0.707106781186548,1.,0.707106781186548,1.),(1.,
0.707106781186548,1.,0.707106781186548,1.,0.707106781186548,1.,0.707106781186548,
1.),(1.,0.707106781186548,1.,0.707106781186548,1.,0.707106781186548,1.,
0.707106781186548,1.),(1.,0.707106781186548,1.,0.707106781186548,1.,0.707106781186548,
1.,0.707106781186548,1.),(1.,0.707106781186548,1.,0.707106781186548,1.,
0.707106781186548,1.,0.707106781186548,1.),(1.,0.707106781186548,1.,0.707106781186548,
1.,0.707106781186548,1.,0.707106781186548,1.),(1.,0.707106781186548,1.,
0.707106781186548,1.,0.707106781186548,1.,0.707106781186548,1.),(1.,0.707106781186548,
1.,0.707106781186548,1.,0.707106781186548,1.,0.707106781186548,1.),(1.,
0.707106781186548,1.,0.707106781186548,1.,0.707106781186548,1.,0.707106781186548,
1.),(1.,0.707106781186548,1.,0.707106781186548,1.,0.707106781186548,1.,
0.707106781186548,1.),(1.,0.707106781186548,1.,0.707106781186548,1.,0.707106781186548,
1.,0.707106781186548,1.),(1.,0.707106781186548,1.,0.707106781186548,1.,
0.707106781186548,1.,0.707106781186548,1.),(1.,0.707106781186548,1.,0.707106781186548,
1.,0.707106781186548,1.,0.707106781186548,1.),(1.,0.707106781186548,1.,
0.707106781186548,1.,0.707106781186548,1.,0.707106781186548,1.),(1.,0.707106781186548,
1.,0.707106781186548,1.,0.707106781186548,1.,0.707106781186548,1.),(1.,
0.707106781186548,1.,0.707106781186548,1.,0.707106781186548,1.,0.707106781186548,
1.),(1.,0.707106781186548,1.,0.707106781186548,1.,0.707106781186548,1.,
0.707106781186548,1.),(1.,0.707106781186548,1.,0.707106781186548,1.,0.707106781186548,
1.,0.707106781186548,1.),(1.,0.707106781186548,1.,0.707106781186548,1.,
0.707106781186548,1.,0.707106781186548,1.),(1.,0.707106781186548,1.,0.707106781186548,
1.,0.707106781186548,1.,0.707106781186548,1.),(1.,0.707106781186548,1.,
0.707106781186548,1.,0.707106781186548,1.,0.707106781186548,1.),(1.,0.707106781186548,
1.,0.707106781186548,1.,0.707106781186548,1.,0.707106781186548,1.),(1.,
0.707106781186548,1.,0.707106781186548,1.,0.707106781186548,1.,0.707106781186548,
1.),(1.,0.707106781186548,1.,0.707106781186548,1.,0.707106781186548,1.,
0.707106781186548,1.),(1.,0.707106781186548,1.,0.707106781186548,1.,0.707106781186548,
1.,0.707106781186548,1.),(1.,0.707106781186548,1.,0.707106781186548,1.,
0.707106781186548,1.,0.707106781186548,1.),(1.,0.707106781186548,1.,0.707106781186548,
1.,0.707106781186548,1.,0.707106781186548,1.),(1.,0.707106781186548,1.,
0.707106781186548,1.,0.707106781186548,1.,0.707106781186548,1.),(1.,0.707106781186548,
1.,0.707106781186548,1.,0.707106781186548,1.,0.707106781186548,1.),(1.,
0.707106781186548,1.,0.707106781186548,1.,0.707106781186548,1.,0.707106781186548,
1.),(1.,0.707106781186548,1.,0.707106781186548,1.,0.707106781186548,1.,
0.707106781186548,1.),(1.,0.707106781186548,1.,0.707106781186548,1.,0.707106781186548,
1.,0.707106781186548,1.),(1.,0.707106781186548,1.,0.707106781186548,1.,
0.707106781186548,1.,0.707106781186548,1.),(1.,0.707106781186548,1.,0.707106781186548,
1.,0.707106781186548,1.,0.707106781186548,1.),(1.,0.707106781186548,1.,
0.707106781186548,1.,0.707106781186548,1.,0.707106781186548,1.),(1.,0.707106781186548,
1.,0.707106781186548,1.,0.707106781186548,1.,0.707106781186548,1.),(1.,
0.707106781186548,1.,0.707106781186548,1.,0.707106781186548,1.,0.707106781186548,
1.),(1.,0.707106781186548,1.,0.707106781186548,1.,0.707106781186548,1.,
0.707106781186548,1.),(1.,0.707106781186548,1.,0.707106781186548,1.,0.707106781186548,
1.,0.707106781186548,1.),(1.,0.707106781186548,1.,0.707106781186548,1.,
0.707106781186548,1.,0.707106781186548,1.),(1.,0.707106781186548,1.,0.707106781186548,
1.,0.707106781186548,1.,0.707106781186548,1.),(1.,0.707106781186548,1.,
0.707106781186548,1.,0.707106781186548,1.,0.707106781186548,1.),(1.,0.707106781186548,
1.,0.707106781186548,1.,0.707106781186548,1.,0.707106781186548,1.),(1.,
0.707106781186548,1.,0.707106781186548,1.,0.707106781186548,1.,0.707106781186548,
1.),(1.,0.707106781186548,1.,0.707106781186548,1.,0.707106781186548,1.,
0.707106781186548,1.),(1.,0.707106781186548,1.,0.707106781186548,1.,0.707106781186548,
1.,0.707106781186548,1.),(1.,0.707106781186548,1.,0.707106781186548,1.,
0.707106781186548,1.,0.707106781186548,1.),(1.,0.707106781186548,1.,0.707106781186548,
1.,0.707106781186548,1.,0.707106781186548,1.),(1.,0.707106781186548,1.,
0.707106781186548,1.,0.707106781186548,1.,0.707106781186548,1.),(1.,0.707106781186548,
1.,0.707106781186548,1.,0.707106781186548,1.,0.707106781186548,1.),(1.,
0.707106781186548,1.,0.707106781186548,1.,0.707106781186548,1.,0.707106781186548,
1.),(1.,0.707106781186548,1.,0.707106781186548,1.,0.707106781186548,1.,
0.707106781186548,1.),(1.,0.707106781186548,1.,0.707106781186548,1.,0.707106781186548,
1.,0.707106781186548,1.),(1.,0.707106781186548,1.,0.707106781186548,1.,
0.707106781186548,1.,0.707106781186548,1.),(1.,0.707106781186548,1.,0.707106781186548,
1.,0.707106781186548,1.,0.707106781186548,1.),(1.,0.707106781186548,1.,
0.707106781186548,1.,0.707106781186548,1.,0.707106781186548,1.),(1.,0.707106781186548,
1.,0.707106781186548,1.,0.707106781186548,1.,0.707106781186548,1.),(1.,
0.707106781186548,1.,0.707106781186548,1.,0.707106781186548,1.,0.707106781186548,
1.),(1.,0.707106781186548,1.,0.707106781186548,1.,0.707106781186548,1.,
0.707106781186548,1.),(1.,0.707106781186548,1.,0.707106781186548,1.,0.707106781186548,
1.,0.707106781186548,1.),(1.,0.707106781186548,1.,0.707106781186548,1.,
0.707106781186548,1.,0.707106781186548,1.),(1.,0.707106781186548,1.,0.707106781186548,
1.,0.707106781186548,1.,0.707106781186548,1.),(1.,0.707106781186548,1.,
0.707106781186548,1.,0.707106781186548,1.,0.707106781186548,1.),(1.,0.707106781186548,
1.,0.707106781186548,1.,0.707106781186548,1.,0.707106781186548,1.),(1.,
0.707106781186548,1.,0.707106781186548,1.,0.707106781186548,1.,0.707106781186548,
1.),(1.,0.707106781186548,1.,0.707106781186548,1.,0.707106781186548,1.,
0.707106781186548,1.),(1.,0.707106781186548,1.,0.707106781186548,1.,0.707106781186548,
1.,0.707106781186548,1.),(1.,0.707106781186548,1.,0.707106781186548,1.,
0.707106781186548,1.,0.707106781186548,1.),(1.,0.707106781186548,1.,0.707106781186548,
1.,0.707106781186548,1.,0.707106781186548,1.),(1.,0.707106781186548,1.,
0.707106781186548,1.,0.707106781186548,1.,0.707106781186548,1.),(1.,0.707106781186548,
1.,0.707106781186548,1.,0.707106781186548,1.,0.707106781186548,1.),(1.,
0.707106781186548,1.,0.707106781186548,1.,0.707106781186548,1.,0.707106781186548,
1.),(1.,0.707106781186548,1.,0.707106781186548,1.,0.707106781186548,1.,
0.707106781186548,1.),(1.,0.707106781186548,1.,0.707106781186548,1.,0.707106781186548,
1.,0.707106781186548,1.),(1.,0.707106781186548,1.,0.707106781186548,1.,
0.707106781186548,1.,0.707106781186548,1.),(1.,0.707106781186548,1.,0.707106781186548,
1.,0.707106781186548,1.,0.707106781186548,1.),(1.,0.707106781186548,1.,
0.707106781186548,1.,0.707106781186548,1.,0.707106781186548,1.),(1.,0.707106781186548,
1.,0.707106781186548,1.,0.707106781186548,1.,0.707106781186548,1.),(1.,
0.707106781186548,1.,0.707106781186548,1.,0.707106781186548,1.,0.707106781186548,
1.),(1.,0.707106781186548,1.,0.707106781186548,1.,0.707106781186548,1.,
0.707106781186548,1.),(1.,0.707106781186548,1.,0.707106781186548,1.,0.707106781186548,
1.,0.707106781186548,1.),(1.,0.707106781186548,1.,0.707106781186548,1.,
0.707106781186548,1.,0.707106781186548,1.),(1.,0.707106781186548,1.,0.707106781186548,
1.,0.707106781186548,1.,0.707106781186548,1.),(1.,0.707106781186548,1.,
0.707106781186548,1.,0.707106781186548,1.,0.707106781186548,1.),(1.,0.707106781186548,
1.,0.707106781186548,1.,0.707106781186548,1.,0.707106781186548,1.),(1.,
0.707106781186548,1.,0.707106781186548,1.,0.707106781186548,1.,0.707106781186548,
1.),(1.,0.707106781186548,1.,0.707106781186548,1.,0.707106781186548,1.,
0.707106781186548,1.),(1.,0.707106781186548,1.,0.707106781186548,1.,0.707106781186548,
1.,0.707106781186548,1.),(1.,0.707106781186548,1.,0.707106781186548,1.,
0.707106781186548,1.,0.707106781186548,1.),(1.,0.707106781186548,1.,0.707106781186548,
1.,0.707106781186548,1.,0.707106781186548,1.),(1.,0.707106781186548,1.,
0.707106781186548,1.,0.707106781186548,1.,0.707106781186548,1.),(1.,0.707106781186548,
1.,0.707106781186548,1.,0.707106781186548,1.,0.707106781186548,1.),(1.,
0.707106781186548,1.,0.707106781186548,1.,0.707106781186548,1.,0.707106781186548,
1.),(1.,0.707106781186548,1.,0.707106781186548,1.,0.707106781186548,1.,
0.707106781186548,1.),(1.,0.707106781186548,1.,0.707106781186548,1.,0.707106781186548,
1.,0.707106781186548,1.),(1.,0.707106781186548,1.,0.707106781186548,1.,
0.707106781186548,1.,0.707106781186548,1.),(1.,0.707106781186548,1.,0.707106781186548,
1.,0.707106781186548,1.,0.707106781186548,1.),(1.,0.707106781186548,1.,
0.707106781186548,1.,0.707106781186548,1.,0.707106781186548,1.),(1.,0.707106781186548,
1.,0.707106781186548,1.,0.707106781186548,1.,0.707106781186548,1.),(1.,
0.707106781186548,1.,0.707106781186548,1.,0.707106781186548,1.,0.707106781186548,
1.),(1.,0.707106781186548,1.,0.707106781186548,1.,0.707106781186548,1.,
0.707106781186548,1.),(1.,0.707106781186548,1.,0.707106781186548,1.,0.707106781186548,
1.,0.707106781186548,1.),(1.,0.707106781186548,1.,0.707106781186548,1.,
0.707106781186548,1.,0.707106781186548,1.),(1.,0.707106781186548,1.,0.707106781186548,
1.,0.707106781186548,1.,0.707106781186548,1.),(1.,0.707106781186548,1.,
0.707106781186548,1.,0.707106781186548,1.,0.707106781186548,1.),(1.,0.707106781186548,
1.,0.707106781186548,1.,0.707106781186548,1.,0.707106781186548,1.),(1.,
0.707106781186548,1.,0.707106781186548,1.,0.707106781186548,1.,0.707106781186548,
1.)))
REPRESENTATION_ITEM('')
SURFACE()
);
#4072=FACE_OUTER_BOUND('',#6502,.T.);
#4073=FACE_OUTER_BOUND('',#6503,.T.);
#4074=FACE_OUTER_BOUND('',#6505,.T.);
#4075=FACE_OUTER_BOUND('',#6506,.T.);
#4076=FACE_OUTER_BOUND('',#6507,.T.);
#4077=FACE_OUTER_BOUND('',#6508,.T.);
#4078=FACE_OUTER_BOUND('',#6510,.T.);
#4079=FACE_OUTER_BOUND('',#6511,.T.);
#4080=FACE_OUTER_BOUND('',#6512,.T.);
#4081=FACE_OUTER_BOUND('',#6513,.T.);
#6502=EDGE_LOOP('',(#34797,#34798,#34799,#34800));
#6503=EDGE_LOOP('',(#34801));
#6504=EDGE_LOOP('',(#34802));
#6505=EDGE_LOOP('',(#34803,#34804,#34805,#34806,#34807));
#6506=EDGE_LOOP('',(#34808,#34809,#34810,#34811,#34812,#34813));
#6507=EDGE_LOOP('',(#34814,#34815,#34816,#34817,#34818));
#6508=EDGE_LOOP('',(#34819));
#6509=EDGE_LOOP('',(#34820));
#6510=EDGE_LOOP('',(#34821,#34822,#34823,#34824));
#6511=EDGE_LOOP('',(#34825,#34826,#34827,#34828,#34829));
#6512=EDGE_LOOP('',(#34830,#34831,#34832,#34833,#34834,#34835));
#6513=EDGE_LOOP('',(#34836,#34837,#34838,#34839,#34840));
#8851=CIRCLE('',#44237,12.);
#8852=CIRCLE('',#44238,12.);
#8853=CIRCLE('',#44240,14.);
#8854=CIRCLE('',#44242,14.);
#8855=CIRCLE('',#44243,14.);
#8856=CIRCLE('',#44244,43.);
#8857=CIRCLE('',#44245,43.);
#8858=CIRCLE('',#44247,43.);
#8859=CIRCLE('',#44249,41.);
#8860=CIRCLE('',#44251,41.);
#8861=CIRCLE('',#44253,40.);
#8862=CIRCLE('',#44254,40.);
#8863=CIRCLE('',#44255,13.5);
#8864=CIRCLE('',#44256,13.5);
#12336=LINE('',#84667,#14830);
#12337=LINE('',#84677,#14831);
#12338=LINE('',#85785,#14832);
#12339=LINE('',#85791,#14833);
#12340=LINE('',#85795,#14834);
#12341=LINE('',#86904,#14835);
#14830=VECTOR('',#54650,12.);
#14831=VECTOR('',#54663,14.);
#14832=VECTOR('',#54672,43.);
#14833=VECTOR('',#54679,41.);
#14834=VECTOR('',#54684,40.5);
#14835=VECTOR('',#54695,12.75);
#18282=VERTEX_POINT('',#84664);
#18283=VERTEX_POINT('',#84666);
#18284=VERTEX_POINT('',#84670);
#18285=VERTEX_POINT('',#84673);
#18286=VERTEX_POINT('',#84674);
#18287=VERTEX_POINT('',#85668);
#18288=VERTEX_POINT('',#85779);
#18289=VERTEX_POINT('',#85783);
#18290=VERTEX_POINT('',#85787);
#18291=VERTEX_POINT('',#85790);
#18292=VERTEX_POINT('',#85794);
#18293=VERTEX_POINT('',#85796);
#18294=VERTEX_POINT('',#86789);
#18295=VERTEX_POINT('',#86900);
#23910=EDGE_CURVE('',#18282,#18282,#8851,.T.);
#23911=EDGE_CURVE('',#18282,#18283,#12336,.T.);
#23912=EDGE_CURVE('',#18283,#18283,#8852,.T.);
#23913=EDGE_CURVE('',#18284,#18284,#8853,.T.);
#23914=EDGE_CURVE('',#18285,#18286,#8854,.T.);
#23915=EDGE_CURVE('',#18286,#18285,#8855,.T.);
#23916=EDGE_CURVE('',#18286,#18284,#12337,.T.);
#23917=EDGE_CURVE('',#18285,#18287,#1929,.T.);
#23918=EDGE_CURVE('',#18288,#18287,#8856,.T.);
#23919=EDGE_CURVE('',#18287,#18288,#8857,.T.);
#23920=EDGE_CURVE('',#18289,#18289,#8858,.T.);
#23921=EDGE_CURVE('',#18289,#18288,#12338,.T.);
#23922=EDGE_CURVE('',#18290,#18290,#8859,.T.);
#23923=EDGE_CURVE('',#18290,#18291,#12339,.T.);
#23924=EDGE_CURVE('',#18291,#18291,#8860,.T.);
#23925=EDGE_CURVE('',#18291,#18292,#12340,.T.);
#23926=EDGE_CURVE('',#18293,#18292,#8861,.T.);
#23927=EDGE_CURVE('',#18292,#18293,#8862,.T.);
#23928=EDGE_CURVE('',#18293,#18294,#1930,.T.);
#23929=EDGE_CURVE('',#18295,#18294,#8863,.T.);
#23930=EDGE_CURVE('',#18294,#18295,#8864,.T.);
#23931=EDGE_CURVE('',#18295,#18282,#12341,.T.);
#34797=ORIENTED_EDGE('',*,*,#23910,.T.);
#34798=ORIENTED_EDGE('',*,*,#23911,.T.);
#34799=ORIENTED_EDGE('',*,*,#23912,.F.);
#34800=ORIENTED_EDGE('',*,*,#23911,.F.);
#34801=ORIENTED_EDGE('',*,*,#23913,.F.);
#34802=ORIENTED_EDGE('',*,*,#23912,.T.);
#34803=ORIENTED_EDGE('',*,*,#23914,.F.);
#34804=ORIENTED_EDGE('',*,*,#23915,.F.);
#34805=ORIENTED_EDGE('',*,*,#23916,.T.);
#34806=ORIENTED_EDGE('',*,*,#23913,.T.);
#34807=ORIENTED_EDGE('',*,*,#23916,.F.);
#34808=ORIENTED_EDGE('',*,*,#23917,.F.);
#34809=ORIENTED_EDGE('',*,*,#23914,.T.);
#34810=ORIENTED_EDGE('',*,*,#23915,.T.);
#34811=ORIENTED_EDGE('',*,*,#23917,.T.);
#34812=ORIENTED_EDGE('',*,*,#23918,.F.);
#34813=ORIENTED_EDGE('',*,*,#23919,.F.);
#34814=ORIENTED_EDGE('',*,*,#23920,.F.);
#34815=ORIENTED_EDGE('',*,*,#23921,.T.);
#34816=ORIENTED_EDGE('',*,*,#23918,.T.);
#34817=ORIENTED_EDGE('',*,*,#23919,.T.);
#34818=ORIENTED_EDGE('',*,*,#23921,.F.);
#34819=ORIENTED_EDGE('',*,*,#23920,.T.);
#34820=ORIENTED_EDGE('',*,*,#23922,.F.);
#34821=ORIENTED_EDGE('',*,*,#23922,.T.);
#34822=ORIENTED_EDGE('',*,*,#23923,.T.);
#34823=ORIENTED_EDGE('',*,*,#23924,.F.);
#34824=ORIENTED_EDGE('',*,*,#23923,.F.);
#34825=ORIENTED_EDGE('',*,*,#23924,.T.);
#34826=ORIENTED_EDGE('',*,*,#23925,.T.);
#34827=ORIENTED_EDGE('',*,*,#23926,.F.);
#34828=ORIENTED_EDGE('',*,*,#23927,.F.);
#34829=ORIENTED_EDGE('',*,*,#23925,.F.);
#34830=ORIENTED_EDGE('',*,*,#23928,.F.);
#34831=ORIENTED_EDGE('',*,*,#23926,.T.);
#34832=ORIENTED_EDGE('',*,*,#23927,.T.);
#34833=ORIENTED_EDGE('',*,*,#23928,.T.);
#34834=ORIENTED_EDGE('',*,*,#23929,.F.);
#34835=ORIENTED_EDGE('',*,*,#23930,.F.);
#34836=ORIENTED_EDGE('',*,*,#23930,.T.);
#34837=ORIENTED_EDGE('',*,*,#23931,.T.);
#34838=ORIENTED_EDGE('',*,*,#23910,.F.);
#34839=ORIENTED_EDGE('',*,*,#23931,.F.);
#34840=ORIENTED_EDGE('',*,*,#23929,.T.);
#37779=CYLINDRICAL_SURFACE('',#44236,12.);
#37780=CYLINDRICAL_SURFACE('',#44241,14.);
#37781=CYLINDRICAL_SURFACE('',#44246,43.);
#37782=CYLINDRICAL_SURFACE('',#44250,41.);
#39875=ADVANCED_FACE('',(#4072),#37779,.F.);
#39876=ADVANCED_FACE('',(#4073,#1073),#1637,.T.);
#39877=ADVANCED_FACE('',(#4074),#37780,.T.);
#39878=ADVANCED_FACE('',(#4075),#1936,.T.);
#39879=ADVANCED_FACE('',(#4076),#37781,.T.);
#39880=ADVANCED_FACE('',(#4077,#1074),#1638,.T.);
#39881=ADVANCED_FACE('',(#4078),#37782,.F.);
#39882=ADVANCED_FACE('',(#4079),#741,.F.);
#39883=ADVANCED_FACE('',(#4080),#1937,.T.);
#39884=ADVANCED_FACE('',(#4081),#742,.F.);
#40355=CLOSED_SHELL('',(#39875,#39876,#39877,#39878,#39879,#39880,#39881,
#39882,#39883,#39884));
#44235=AXIS2_PLACEMENT_3D('',#84662,#54644,#54645);
#44236=AXIS2_PLACEMENT_3D('',#84663,#54646,#54647);
#44237=AXIS2_PLACEMENT_3D('',#84665,#54648,#54649);
#44238=AXIS2_PLACEMENT_3D('',#84668,#54651,#54652);
#44239=AXIS2_PLACEMENT_3D('',#84669,#54653,#54654);
#44240=AXIS2_PLACEMENT_3D('',#84671,#54655,#54656);
#44241=AXIS2_PLACEMENT_3D('',#84672,#54657,#54658);
#44242=AXIS2_PLACEMENT_3D('',#84675,#54659,#54660);
#44243=AXIS2_PLACEMENT_3D('',#84676,#54661,#54662);
#44244=AXIS2_PLACEMENT_3D('',#85780,#54664,#54665);
#44245=AXIS2_PLACEMENT_3D('',#85781,#54666,#54667);
#44246=AXIS2_PLACEMENT_3D('',#85782,#54668,#54669);
#44247=AXIS2_PLACEMENT_3D('',#85784,#54670,#54671);
#44248=AXIS2_PLACEMENT_3D('',#85786,#54673,#54674);
#44249=AXIS2_PLACEMENT_3D('',#85788,#54675,#54676);
#44250=AXIS2_PLACEMENT_3D('',#85789,#54677,#54678);
#44251=AXIS2_PLACEMENT_3D('',#85792,#54680,#54681);
#44252=AXIS2_PLACEMENT_3D('',#85793,#54682,#54683);
#44253=AXIS2_PLACEMENT_3D('',#85797,#54685,#54686);
#44254=AXIS2_PLACEMENT_3D('',#85798,#54687,#54688);
#44255=AXIS2_PLACEMENT_3D('',#86901,#54689,#54690);
#44256=AXIS2_PLACEMENT_3D('',#86902,#54691,#54692);
#44257=AXIS2_PLACEMENT_3D('',#86903,#54693,#54694);
#54644=DIRECTION('axis',(0.,0.,1.));
#54645=DIRECTION('refdir',(1.,0.,0.));
#54646=DIRECTION('center_axis',(1.,0.,0.));
#54647=DIRECTION('ref_axis',(0.,1.,0.));
#54648=DIRECTION('center_axis',(1.,0.,0.));
#54649=DIRECTION('ref_axis',(0.,0.,-1.));
#54650=DIRECTION('',(-1.,0.,0.));
#54651=DIRECTION('center_axis',(1.,0.,0.));
#54652=DIRECTION('ref_axis',(0.,0.,-1.));
#54653=DIRECTION('center_axis',(-1.,0.,0.));
#54654=DIRECTION('ref_axis',(0.,0.,1.));
#54655=DIRECTION('center_axis',(1.,0.,0.));
#54656=DIRECTION('ref_axis',(0.,0.,-1.));
#54657=DIRECTION('center_axis',(1.,0.,0.));
#54658=DIRECTION('ref_axis',(0.,1.,0.));
#54659=DIRECTION('center_axis',(1.,0.,0.));
#54660=DIRECTION('ref_axis',(0.,0.,-1.));
#54661=DIRECTION('center_axis',(1.,0.,0.));
#54662=DIRECTION('ref_axis',(0.,0.,-1.));
#54663=DIRECTION('',(-1.,0.,0.));
#54664=DIRECTION('center_axis',(1.,0.,0.));
#54665=DIRECTION('ref_axis',(0.,0.,-1.));
#54666=DIRECTION('center_axis',(1.,0.,0.));
#54667=DIRECTION('ref_axis',(0.,0.,-1.));
#54668=DIRECTION('center_axis',(1.,0.,0.));
#54669=DIRECTION('ref_axis',(0.,1.,0.));
#54670=DIRECTION('center_axis',(1.,0.,0.));
#54671=DIRECTION('ref_axis',(0.,0.,-1.));
#54672=DIRECTION('',(-1.,0.,0.));
#54673=DIRECTION('center_axis',(1.,0.,0.));
#54674=DIRECTION('ref_axis',(0.,0.,-1.));
#54675=DIRECTION('center_axis',(1.,0.,0.));
#54676=DIRECTION('ref_axis',(0.,0.,-1.));
#54677=DIRECTION('center_axis',(1.,0.,0.));
#54678=DIRECTION('ref_axis',(0.,1.,0.));
#54679=DIRECTION('',(-1.,0.,0.));
#54680=DIRECTION('center_axis',(1.,0.,0.));
#54681=DIRECTION('ref_axis',(0.,0.,-1.));
#54682=DIRECTION('center_axis',(1.,0.,0.));
#54683=DIRECTION('ref_axis',(0.,1.,0.));
#54684=DIRECTION('',(-0.768221279597389,0.640184399664464,7.83999775913156E-17));
#54685=DIRECTION('center_axis',(1.,0.,0.));
#54686=DIRECTION('ref_axis',(0.,0.,-1.));
#54687=DIRECTION('center_axis',(1.,0.,0.));
#54688=DIRECTION('ref_axis',(0.,0.,-1.));
#54689=DIRECTION('center_axis',(1.,0.,0.));
#54690=DIRECTION('ref_axis',(0.,0.,-1.));
#54691=DIRECTION('center_axis',(1.,0.,0.));
#54692=DIRECTION('ref_axis',(0.,0.,-1.));
#54693=DIRECTION('center_axis',(1.,0.,0.));
#54694=DIRECTION('ref_axis',(0.,1.,0.));
#54695=DIRECTION('',(-0.554700196225234,0.83205029433784,1.01896772969045E-16));
#84662=CARTESIAN_POINT('',(0.,0.,0.));
#84663=CARTESIAN_POINT('Origin',(422.5,0.,0.));
#84664=CARTESIAN_POINT('',(430.,-12.,-1.46957615897682E-15));
#84665=CARTESIAN_POINT('Origin',(430.,0.,0.));
#84666=CARTESIAN_POINT('',(415.,-12.,-1.46957615897682E-15));
#84667=CARTESIAN_POINT('',(422.5,-12.,-1.46957615897682E-15));
#84668=CARTESIAN_POINT('Origin',(415.,0.,0.));
#84669=CARTESIAN_POINT('Origin',(415.,14.,0.));
#84670=CARTESIAN_POINT('',(415.,-14.,-1.71450551880629E-15));
#84671=CARTESIAN_POINT('Origin',(415.,0.,0.));
#84672=CARTESIAN_POINT('Origin',(422.5,0.,0.));
#84673=CARTESIAN_POINT('',(430.,14.,0.));
#84674=CARTESIAN_POINT('',(430.,-14.,-1.71450551880629E-15));
#84675=CARTESIAN_POINT('Origin',(430.,0.,0.));
#84676=CARTESIAN_POINT('Origin',(430.,0.,0.));
#84677=CARTESIAN_POINT('',(422.5,-14.,-1.71450551880629E-15));
#84678=CARTESIAN_POINT('Ctrl Pts',(498.,43.,0.));
#84679=CARTESIAN_POINT('Ctrl Pts',(498.,43.,43.));
#84680=CARTESIAN_POINT('Ctrl Pts',(498.,0.,43.));
#84681=CARTESIAN_POINT('Ctrl Pts',(498.,-43.,43.));
#84682=CARTESIAN_POINT('Ctrl Pts',(498.,-43.,0.));
#84683=CARTESIAN_POINT('Ctrl Pts',(498.,-43.,-43.));
#84684=CARTESIAN_POINT('Ctrl Pts',(498.,0.,-43.));
#84685=CARTESIAN_POINT('Ctrl Pts',(498.,43.,-43.));
#84686=CARTESIAN_POINT('Ctrl Pts',(498.,43.,0.));
#84687=CARTESIAN_POINT('Ctrl Pts',(497.919875683486,42.8463072547191,0.));
#84688=CARTESIAN_POINT('Ctrl Pts',(497.919875683486,42.846307254719,42.846307254719));
#84689=CARTESIAN_POINT('Ctrl Pts',(497.919875683486,0.,42.8463072547191));
#84690=CARTESIAN_POINT('Ctrl Pts',(497.919875683486,-42.846307254719,42.846307254719));
#84691=CARTESIAN_POINT('Ctrl Pts',(497.919875683486,-42.8463072547191,0.));
#84692=CARTESIAN_POINT('Ctrl Pts',(497.919875683486,-42.846307254719,-42.846307254719));
#84693=CARTESIAN_POINT('Ctrl Pts',(497.919875683486,0.,-42.8463072547191));
#84694=CARTESIAN_POINT('Ctrl Pts',(497.919875683486,42.846307254719,-42.846307254719));
#84695=CARTESIAN_POINT('Ctrl Pts',(497.919875683486,42.8463072547191,0.));
#84696=CARTESIAN_POINT('Ctrl Pts',(497.754018276443,42.5357609366511,0.));
#84697=CARTESIAN_POINT('Ctrl Pts',(497.754018276443,42.5357609366511,42.5357609366511));
#84698=CARTESIAN_POINT('Ctrl Pts',(497.754018276443,0.,42.5357609366511));
#84699=CARTESIAN_POINT('Ctrl Pts',(497.754018276443,-42.5357609366511,42.5357609366511));
#84700=CARTESIAN_POINT('Ctrl Pts',(497.754018276443,-42.5357609366511,0.));
#84701=CARTESIAN_POINT('Ctrl Pts',(497.754018276443,-42.5357609366511,-42.5357609366511));
#84702=CARTESIAN_POINT('Ctrl Pts',(497.754018276443,0.,-42.5357609366511));
#84703=CARTESIAN_POINT('Ctrl Pts',(497.754018276443,42.5357609366511,-42.5357609366511));
#84704=CARTESIAN_POINT('Ctrl Pts',(497.754018276443,42.5357609366511,0.));
#84705=CARTESIAN_POINT('Ctrl Pts',(497.488406157359,42.0604608545242,0.));
#84706=CARTESIAN_POINT('Ctrl Pts',(497.488406157359,42.0604608545242,42.0604608545242));
#84707=CARTESIAN_POINT('Ctrl Pts',(497.488406157359,0.,42.0604608545242));
#84708=CARTESIAN_POINT('Ctrl Pts',(497.488406157359,-42.0604608545242,42.0604608545242));
#84709=CARTESIAN_POINT('Ctrl Pts',(497.488406157359,-42.0604608545242,0.));
#84710=CARTESIAN_POINT('Ctrl Pts',(497.488406157359,-42.0604608545242,-42.0604608545242));
#84711=CARTESIAN_POINT('Ctrl Pts',(497.488406157359,0.,-42.0604608545242));
#84712=CARTESIAN_POINT('Ctrl Pts',(497.488406157359,42.0604608545242,-42.0604608545242));
#84713=CARTESIAN_POINT('Ctrl Pts',(497.488406157359,42.0604608545242,0.));
#84714=CARTESIAN_POINT('Ctrl Pts',(497.100596959865,41.4077471164017,0.));
#84715=CARTESIAN_POINT('Ctrl Pts',(497.100596959865,41.4077471164017,41.4077471164017));
#84716=CARTESIAN_POINT('Ctrl Pts',(497.100596959865,0.,41.4077471164017));
#84717=CARTESIAN_POINT('Ctrl Pts',(497.100596959865,-41.4077471164017,41.4077471164017));
#84718=CARTESIAN_POINT('Ctrl Pts',(497.100596959865,-41.4077471164017,0.));
#84719=CARTESIAN_POINT('Ctrl Pts',(497.100596959865,-41.4077471164017,-41.4077471164017));
#84720=CARTESIAN_POINT('Ctrl Pts',(497.100596959865,0.,-41.4077471164017));
#84721=CARTESIAN_POINT('Ctrl Pts',(497.100596959865,41.4077471164017,-41.4077471164017));
#84722=CARTESIAN_POINT('Ctrl Pts',(497.100596959865,41.4077471164017,0.));
#84723=CARTESIAN_POINT('Ctrl Pts',(496.560639185004,40.5647779062035,0.));
#84724=CARTESIAN_POINT('Ctrl Pts',(496.560639185004,40.5647779062034,40.5647779062034));
#84725=CARTESIAN_POINT('Ctrl Pts',(496.560639185004,0.,40.5647779062035));
#84726=CARTESIAN_POINT('Ctrl Pts',(496.560639185004,-40.5647779062034,40.5647779062034));
#84727=CARTESIAN_POINT('Ctrl Pts',(496.560639185004,-40.5647779062035,0.));
#84728=CARTESIAN_POINT('Ctrl Pts',(496.560639185004,-40.5647779062034,-40.5647779062034));
#84729=CARTESIAN_POINT('Ctrl Pts',(496.560639185004,0.,-40.5647779062035));
#84730=CARTESIAN_POINT('Ctrl Pts',(496.560639185004,40.5647779062034,-40.5647779062034));
#84731=CARTESIAN_POINT('Ctrl Pts',(496.560639185004,40.5647779062035,0.));
#84732=CARTESIAN_POINT('Ctrl Pts',(495.968194348492,39.7081288650878,0.));
#84733=CARTESIAN_POINT('Ctrl Pts',(495.968194348492,39.7081288650878,39.7081288650878));
#84734=CARTESIAN_POINT('Ctrl Pts',(495.968194348492,0.,39.7081288650878));
#84735=CARTESIAN_POINT('Ctrl Pts',(495.968194348492,-39.7081288650878,39.7081288650878));
#84736=CARTESIAN_POINT('Ctrl Pts',(495.968194348492,-39.7081288650878,0.));
#84737=CARTESIAN_POINT('Ctrl Pts',(495.968194348492,-39.7081288650878,-39.7081288650878));
#84738=CARTESIAN_POINT('Ctrl Pts',(495.968194348492,0.,-39.7081288650878));
#84739=CARTESIAN_POINT('Ctrl Pts',(495.968194348492,39.7081288650878,-39.7081288650878));
#84740=CARTESIAN_POINT('Ctrl Pts',(495.968194348492,39.7081288650878,0.));
#84741=CARTESIAN_POINT('Ctrl Pts',(495.328808380576,38.8651538927084,0.));
#84742=CARTESIAN_POINT('Ctrl Pts',(495.328808380576,38.8651538927084,38.8651538927084));
#84743=CARTESIAN_POINT('Ctrl Pts',(495.328808380576,0.,38.8651538927084));
#84744=CARTESIAN_POINT('Ctrl Pts',(495.328808380576,-38.8651538927084,38.8651538927084));
#84745=CARTESIAN_POINT('Ctrl Pts',(495.328808380576,-38.8651538927084,0.));
#84746=CARTESIAN_POINT('Ctrl Pts',(495.328808380576,-38.8651538927084,-38.8651538927084));
#84747=CARTESIAN_POINT('Ctrl Pts',(495.328808380576,0.,-38.8651538927084));
#84748=CARTESIAN_POINT('Ctrl Pts',(495.328808380576,38.8651538927084,-38.8651538927084));
#84749=CARTESIAN_POINT('Ctrl Pts',(495.328808380576,38.8651538927084,0.));
#84750=CARTESIAN_POINT('Ctrl Pts',(494.651570478316,38.080336648354,0.));
#84751=CARTESIAN_POINT('Ctrl Pts',(494.651570478316,38.080336648354,38.080336648354));
#84752=CARTESIAN_POINT('Ctrl Pts',(494.651570478316,0.,38.080336648354));
#84753=CARTESIAN_POINT('Ctrl Pts',(494.651570478316,-38.080336648354,38.080336648354));
#84754=CARTESIAN_POINT('Ctrl Pts',(494.651570478316,-38.080336648354,0.));
#84755=CARTESIAN_POINT('Ctrl Pts',(494.651570478316,-38.080336648354,-38.080336648354));
#84756=CARTESIAN_POINT('Ctrl Pts',(494.651570478316,0.,-38.080336648354));
#84757=CARTESIAN_POINT('Ctrl Pts',(494.651570478316,38.080336648354,-38.080336648354));
#84758=CARTESIAN_POINT('Ctrl Pts',(494.651570478316,38.080336648354,0.));
#84759=CARTESIAN_POINT('Ctrl Pts',(493.950613427123,37.4232171946361,0.));
#84760=CARTESIAN_POINT('Ctrl Pts',(493.950613427123,37.4232171946361,37.4232171946361));
#84761=CARTESIAN_POINT('Ctrl Pts',(493.950613427123,0.,37.4232171946361));
#84762=CARTESIAN_POINT('Ctrl Pts',(493.950613427123,-37.4232171946361,37.4232171946361));
#84763=CARTESIAN_POINT('Ctrl Pts',(493.950613427123,-37.4232171946361,0.));
#84764=CARTESIAN_POINT('Ctrl Pts',(493.950613427123,-37.4232171946361,-37.4232171946361));
#84765=CARTESIAN_POINT('Ctrl Pts',(493.950613427123,0.,-37.4232171946361));
#84766=CARTESIAN_POINT('Ctrl Pts',(493.950613427123,37.4232171946361,-37.4232171946361));
#84767=CARTESIAN_POINT('Ctrl Pts',(493.950613427123,37.4232171946361,0.));
#84768=CARTESIAN_POINT('Ctrl Pts',(493.243601186251,36.978223468014,0.));
#84769=CARTESIAN_POINT('Ctrl Pts',(493.243601186251,36.978223468014,36.978223468014));
#84770=CARTESIAN_POINT('Ctrl Pts',(493.243601186251,0.,36.978223468014));
#84771=CARTESIAN_POINT('Ctrl Pts',(493.243601186251,-36.978223468014,36.978223468014));
#84772=CARTESIAN_POINT('Ctrl Pts',(493.243601186251,-36.978223468014,0.));
#84773=CARTESIAN_POINT('Ctrl Pts',(493.243601186251,-36.978223468014,-36.978223468014));
#84774=CARTESIAN_POINT('Ctrl Pts',(493.243601186251,0.,-36.978223468014));
#84775=CARTESIAN_POINT('Ctrl Pts',(493.243601186251,36.978223468014,-36.978223468014));
#84776=CARTESIAN_POINT('Ctrl Pts',(493.243601186251,36.978223468014,0.));
#84777=CARTESIAN_POINT('Ctrl Pts',(492.547316355638,36.8168662015777,0.));
#84778=CARTESIAN_POINT('Ctrl Pts',(492.547316355638,36.8168662015777,36.8168662015777));
#84779=CARTESIAN_POINT('Ctrl Pts',(492.547316355638,0.,36.8168662015777));
#84780=CARTESIAN_POINT('Ctrl Pts',(492.547316355638,-36.8168662015777,36.8168662015777));
#84781=CARTESIAN_POINT('Ctrl Pts',(492.547316355638,-36.8168662015777,0.));
#84782=CARTESIAN_POINT('Ctrl Pts',(492.547316355638,-36.8168662015777,-36.8168662015777));
#84783=CARTESIAN_POINT('Ctrl Pts',(492.547316355638,0.,-36.8168662015777));
#84784=CARTESIAN_POINT('Ctrl Pts',(492.547316355638,36.8168662015777,-36.8168662015777));
#84785=CARTESIAN_POINT('Ctrl Pts',(492.547316355638,36.8168662015777,0.));
#84786=CARTESIAN_POINT('Ctrl Pts',(491.874247942463,36.9763167796813,0.));
#84787=CARTESIAN_POINT('Ctrl Pts',(491.874247942463,36.9763167796813,36.9763167796813));
#84788=CARTESIAN_POINT('Ctrl Pts',(491.874247942463,0.,36.9763167796813));
#84789=CARTESIAN_POINT('Ctrl Pts',(491.874247942463,-36.9763167796813,36.9763167796813));
#84790=CARTESIAN_POINT('Ctrl Pts',(491.874247942463,-36.9763167796813,0.));
#84791=CARTESIAN_POINT('Ctrl Pts',(491.874247942463,-36.9763167796813,-36.9763167796813));
#84792=CARTESIAN_POINT('Ctrl Pts',(491.874247942463,0.,-36.9763167796813));
#84793=CARTESIAN_POINT('Ctrl Pts',(491.874247942463,36.9763167796813,-36.9763167796813));
#84794=CARTESIAN_POINT('Ctrl Pts',(491.874247942463,36.9763167796813,0.));
#84795=CARTESIAN_POINT('Ctrl Pts',(491.228327780497,37.4320007627789,0.));
#84796=CARTESIAN_POINT('Ctrl Pts',(491.228327780497,37.4320007627789,37.4320007627789));
#84797=CARTESIAN_POINT('Ctrl Pts',(491.228327780497,0.,37.4320007627789));
#84798=CARTESIAN_POINT('Ctrl Pts',(491.228327780497,-37.4320007627789,37.4320007627789));
#84799=CARTESIAN_POINT('Ctrl Pts',(491.228327780497,-37.4320007627789,0.));
#84800=CARTESIAN_POINT('Ctrl Pts',(491.228327780497,-37.4320007627789,-37.4320007627789));
#84801=CARTESIAN_POINT('Ctrl Pts',(491.228327780497,0.,-37.4320007627789));
#84802=CARTESIAN_POINT('Ctrl Pts',(491.228327780497,37.4320007627789,-37.4320007627789));
#84803=CARTESIAN_POINT('Ctrl Pts',(491.228327780497,37.4320007627789,0.));
#84804=CARTESIAN_POINT('Ctrl Pts',(490.602330907815,38.0826279556129,0.));
#84805=CARTESIAN_POINT('Ctrl Pts',(490.602330907815,38.0826279556129,38.0826279556129));
#84806=CARTESIAN_POINT('Ctrl Pts',(490.602330907815,0.,38.0826279556129));
#84807=CARTESIAN_POINT('Ctrl Pts',(490.602330907815,-38.0826279556129,38.0826279556129));
#84808=CARTESIAN_POINT('Ctrl Pts',(490.602330907815,-38.0826279556129,0.));
#84809=CARTESIAN_POINT('Ctrl Pts',(490.602330907815,-38.0826279556129,-38.0826279556129));
#84810=CARTESIAN_POINT('Ctrl Pts',(490.602330907815,0.,-38.0826279556129));
#84811=CARTESIAN_POINT('Ctrl Pts',(490.602330907815,38.0826279556129,-38.0826279556129));
#84812=CARTESIAN_POINT('Ctrl Pts',(490.602330907815,38.0826279556129,0.));
#84813=CARTESIAN_POINT('Ctrl Pts',(489.982486856253,38.7890664196497,0.));
#84814=CARTESIAN_POINT('Ctrl Pts',(489.982486856253,38.7890664196497,38.7890664196497));
#84815=CARTESIAN_POINT('Ctrl Pts',(489.982486856253,0.,38.7890664196497));
#84816=CARTESIAN_POINT('Ctrl Pts',(489.982486856253,-38.7890664196497,38.7890664196497));
#84817=CARTESIAN_POINT('Ctrl Pts',(489.982486856253,-38.7890664196497,0.));
#84818=CARTESIAN_POINT('Ctrl Pts',(489.982486856253,-38.7890664196497,-38.7890664196497));
#84819=CARTESIAN_POINT('Ctrl Pts',(489.982486856253,0.,-38.7890664196497));
#84820=CARTESIAN_POINT('Ctrl Pts',(489.982486856253,38.7890664196497,-38.7890664196497));
#84821=CARTESIAN_POINT('Ctrl Pts',(489.982486856253,38.7890664196497,0.));
#84822=CARTESIAN_POINT('Ctrl Pts',(489.35228088106,39.4079242082379,0.));
#84823=CARTESIAN_POINT('Ctrl Pts',(489.35228088106,39.4079242082379,39.4079242082379));
#84824=CARTESIAN_POINT('Ctrl Pts',(489.35228088106,0.,39.4079242082379));
#84825=CARTESIAN_POINT('Ctrl Pts',(489.35228088106,-39.4079242082379,39.4079242082379));
#84826=CARTESIAN_POINT('Ctrl Pts',(489.35228088106,-39.4079242082379,0.));
#84827=CARTESIAN_POINT('Ctrl Pts',(489.35228088106,-39.4079242082379,-39.4079242082379));
#84828=CARTESIAN_POINT('Ctrl Pts',(489.35228088106,0.,-39.4079242082379));
#84829=CARTESIAN_POINT('Ctrl Pts',(489.35228088106,39.4079242082379,-39.4079242082379));
#84830=CARTESIAN_POINT('Ctrl Pts',(489.35228088106,39.4079242082379,0.));
#84831=CARTESIAN_POINT('Ctrl Pts',(488.696302016509,39.8235950753685,0.));
#84832=CARTESIAN_POINT('Ctrl Pts',(488.696302016509,39.8235950753685,39.8235950753685));
#84833=CARTESIAN_POINT('Ctrl Pts',(488.696302016509,0.,39.8235950753685));
#84834=CARTESIAN_POINT('Ctrl Pts',(488.696302016509,-39.8235950753685,39.8235950753685));
#84835=CARTESIAN_POINT('Ctrl Pts',(488.696302016509,-39.8235950753685,0.));
#84836=CARTESIAN_POINT('Ctrl Pts',(488.696302016509,-39.8235950753685,-39.8235950753685));
#84837=CARTESIAN_POINT('Ctrl Pts',(488.696302016509,0.,-39.8235950753685));
#84838=CARTESIAN_POINT('Ctrl Pts',(488.696302016509,39.8235950753685,-39.8235950753685));
#84839=CARTESIAN_POINT('Ctrl Pts',(488.696302016509,39.8235950753685,0.));
#84840=CARTESIAN_POINT('Ctrl Pts',(488.00470898085,39.9896159368436,0.));
#84841=CARTESIAN_POINT('Ctrl Pts',(488.00470898085,39.9896159368436,39.9896159368436));
#84842=CARTESIAN_POINT('Ctrl Pts',(488.00470898085,0.,39.9896159368436));
#84843=CARTESIAN_POINT('Ctrl Pts',(488.00470898085,-39.9896159368436,39.9896159368436));
#84844=CARTESIAN_POINT('Ctrl Pts',(488.00470898085,-39.9896159368436,0.));
#84845=CARTESIAN_POINT('Ctrl Pts',(488.00470898085,-39.9896159368436,-39.9896159368436));
#84846=CARTESIAN_POINT('Ctrl Pts',(488.00470898085,0.,-39.9896159368436));
#84847=CARTESIAN_POINT('Ctrl Pts',(488.00470898085,39.9896159368436,-39.9896159368436));
#84848=CARTESIAN_POINT('Ctrl Pts',(488.00470898085,39.9896159368436,0.));
#84849=CARTESIAN_POINT('Ctrl Pts',(487.275021660065,39.9329323721432,0.));
#84850=CARTESIAN_POINT('Ctrl Pts',(487.275021660065,39.9329323721432,39.9329323721432));
#84851=CARTESIAN_POINT('Ctrl Pts',(487.275021660065,0.,39.9329323721432));
#84852=CARTESIAN_POINT('Ctrl Pts',(487.275021660065,-39.9329323721432,39.9329323721432));
#84853=CARTESIAN_POINT('Ctrl Pts',(487.275021660065,-39.9329323721432,0.));
#84854=CARTESIAN_POINT('Ctrl Pts',(487.275021660065,-39.9329323721432,-39.9329323721432));
#84855=CARTESIAN_POINT('Ctrl Pts',(487.275021660065,0.,-39.9329323721432));
#84856=CARTESIAN_POINT('Ctrl Pts',(487.275021660065,39.9329323721432,-39.9329323721432));
#84857=CARTESIAN_POINT('Ctrl Pts',(487.275021660065,39.9329323721432,0.));
#84858=CARTESIAN_POINT('Ctrl Pts',(486.510844647409,39.7133643175418,0.));
#84859=CARTESIAN_POINT('Ctrl Pts',(486.510844647409,39.7133643175418,39.7133643175418));
#84860=CARTESIAN_POINT('Ctrl Pts',(486.510844647409,0.,39.7133643175418));
#84861=CARTESIAN_POINT('Ctrl Pts',(486.510844647409,-39.7133643175418,39.7133643175418));
#84862=CARTESIAN_POINT('Ctrl Pts',(486.510844647409,-39.7133643175418,0.));
#84863=CARTESIAN_POINT('Ctrl Pts',(486.510844647409,-39.7133643175418,-39.7133643175418));
#84864=CARTESIAN_POINT('Ctrl Pts',(486.510844647409,0.,-39.7133643175418));
#84865=CARTESIAN_POINT('Ctrl Pts',(486.510844647409,39.7133643175418,-39.7133643175418));
#84866=CARTESIAN_POINT('Ctrl Pts',(486.510844647409,39.7133643175418,0.));
#84867=CARTESIAN_POINT('Ctrl Pts',(485.721282963476,39.3972368241277,0.));
#84868=CARTESIAN_POINT('Ctrl Pts',(485.721282963476,39.3972368241277,39.3972368241277));
#84869=CARTESIAN_POINT('Ctrl Pts',(485.721282963476,0.,39.3972368241277));
#84870=CARTESIAN_POINT('Ctrl Pts',(485.721282963476,-39.3972368241277,39.3972368241277));
#84871=CARTESIAN_POINT('Ctrl Pts',(485.721282963476,-39.3972368241277,0.));
#84872=CARTESIAN_POINT('Ctrl Pts',(485.721282963476,-39.3972368241277,-39.3972368241277));
#84873=CARTESIAN_POINT('Ctrl Pts',(485.721282963476,0.,-39.3972368241277));
#84874=CARTESIAN_POINT('Ctrl Pts',(485.721282963476,39.3972368241277,-39.3972368241277));
#84875=CARTESIAN_POINT('Ctrl Pts',(485.721282963476,39.3972368241277,0.));
#84876=CARTESIAN_POINT('Ctrl Pts',(484.9203435101,39.0198093895239,0.));
#84877=CARTESIAN_POINT('Ctrl Pts',(484.9203435101,39.0198093895238,39.0198093895238));
#84878=CARTESIAN_POINT('Ctrl Pts',(484.9203435101,0.,39.0198093895239));
#84879=CARTESIAN_POINT('Ctrl Pts',(484.9203435101,-39.0198093895238,39.0198093895238));
#84880=CARTESIAN_POINT('Ctrl Pts',(484.9203435101,-39.0198093895239,0.));
#84881=CARTESIAN_POINT('Ctrl Pts',(484.9203435101,-39.0198093895238,-39.0198093895238));
#84882=CARTESIAN_POINT('Ctrl Pts',(484.9203435101,0.,-39.0198093895239));
#84883=CARTESIAN_POINT('Ctrl Pts',(484.9203435101,39.0198093895238,-39.0198093895238));
#84884=CARTESIAN_POINT('Ctrl Pts',(484.9203435101,39.0198093895239,0.));
#84885=CARTESIAN_POINT('Ctrl Pts',(484.125459941715,38.5707804214382,0.));
#84886=CARTESIAN_POINT('Ctrl Pts',(484.125459941715,38.5707804214382,38.5707804214382));
#84887=CARTESIAN_POINT('Ctrl Pts',(484.125459941715,0.,38.5707804214382));
#84888=CARTESIAN_POINT('Ctrl Pts',(484.125459941715,-38.5707804214382,38.5707804214382));
#84889=CARTESIAN_POINT('Ctrl Pts',(484.125459941715,-38.5707804214382,0.));
#84890=CARTESIAN_POINT('Ctrl Pts',(484.125459941715,-38.5707804214382,-38.5707804214382));
#84891=CARTESIAN_POINT('Ctrl Pts',(484.125459941715,0.,-38.5707804214382));
#84892=CARTESIAN_POINT('Ctrl Pts',(484.125459941715,38.5707804214382,-38.5707804214382));
#84893=CARTESIAN_POINT('Ctrl Pts',(484.125459941715,38.5707804214382,0.));
#84894=CARTESIAN_POINT('Ctrl Pts',(483.354083971076,38.0181299396445,0.));
#84895=CARTESIAN_POINT('Ctrl Pts',(483.354083971076,38.0181299396445,38.0181299396445));
#84896=CARTESIAN_POINT('Ctrl Pts',(483.354083971076,0.,38.0181299396445));
#84897=CARTESIAN_POINT('Ctrl Pts',(483.354083971076,-38.0181299396445,38.0181299396445));
#84898=CARTESIAN_POINT('Ctrl Pts',(483.354083971076,-38.0181299396445,0.));
#84899=CARTESIAN_POINT('Ctrl Pts',(483.354083971076,-38.0181299396445,-38.0181299396445));
#84900=CARTESIAN_POINT('Ctrl Pts',(483.354083971076,0.,-38.0181299396445));
#84901=CARTESIAN_POINT('Ctrl Pts',(483.354083971076,38.0181299396445,-38.0181299396445));
#84902=CARTESIAN_POINT('Ctrl Pts',(483.354083971076,38.0181299396445,0.));
#84903=CARTESIAN_POINT('Ctrl Pts',(482.620675064127,37.3238846021003,0.));
#84904=CARTESIAN_POINT('Ctrl Pts',(482.620675064127,37.3238846021003,37.3238846021003));
#84905=CARTESIAN_POINT('Ctrl Pts',(482.620675064127,0.,37.3238846021003));
#84906=CARTESIAN_POINT('Ctrl Pts',(482.620675064127,-37.3238846021003,37.3238846021003));
#84907=CARTESIAN_POINT('Ctrl Pts',(482.620675064127,-37.3238846021003,0.));
#84908=CARTESIAN_POINT('Ctrl Pts',(482.620675064127,-37.3238846021003,-37.3238846021003));
#84909=CARTESIAN_POINT('Ctrl Pts',(482.620675064127,0.,-37.3238846021003));
#84910=CARTESIAN_POINT('Ctrl Pts',(482.620675064127,37.3238846021003,-37.3238846021003));
#84911=CARTESIAN_POINT('Ctrl Pts',(482.620675064127,37.3238846021003,0.));
#84912=CARTESIAN_POINT('Ctrl Pts',(481.933610981183,36.4627634902989,0.));
#84913=CARTESIAN_POINT('Ctrl Pts',(481.933610981183,36.4627634902988,36.4627634902988));
#84914=CARTESIAN_POINT('Ctrl Pts',(481.933610981183,0.,36.4627634902989));
#84915=CARTESIAN_POINT('Ctrl Pts',(481.933610981183,-36.4627634902988,36.4627634902988));
#84916=CARTESIAN_POINT('Ctrl Pts',(481.933610981183,-36.4627634902989,0.));
#84917=CARTESIAN_POINT('Ctrl Pts',(481.933610981183,-36.4627634902988,-36.4627634902988));
#84918=CARTESIAN_POINT('Ctrl Pts',(481.933610981183,0.,-36.4627634902989));
#84919=CARTESIAN_POINT('Ctrl Pts',(481.933610981183,36.4627634902988,-36.4627634902988));
#84920=CARTESIAN_POINT('Ctrl Pts',(481.933610981183,36.4627634902989,0.));
#84921=CARTESIAN_POINT('Ctrl Pts',(481.291935021843,35.4403955291427,0.));
#84922=CARTESIAN_POINT('Ctrl Pts',(481.291935021843,35.4403955291427,35.4403955291427));
#84923=CARTESIAN_POINT('Ctrl Pts',(481.291935021843,0.,35.4403955291427));
#84924=CARTESIAN_POINT('Ctrl Pts',(481.291935021843,-35.4403955291427,35.4403955291427));
#84925=CARTESIAN_POINT('Ctrl Pts',(481.291935021843,-35.4403955291427,0.));
#84926=CARTESIAN_POINT('Ctrl Pts',(481.291935021843,-35.4403955291427,-35.4403955291427));
#84927=CARTESIAN_POINT('Ctrl Pts',(481.291935021843,0.,-35.4403955291427));
#84928=CARTESIAN_POINT('Ctrl Pts',(481.291935021843,35.4403955291427,-35.4403955291427));
#84929=CARTESIAN_POINT('Ctrl Pts',(481.291935021843,35.4403955291427,0.));
#84930=CARTESIAN_POINT('Ctrl Pts',(480.682720968628,34.3094577320604,0.));
#84931=CARTESIAN_POINT('Ctrl Pts',(480.682720968628,34.3094577320603,34.3094577320603));
#84932=CARTESIAN_POINT('Ctrl Pts',(480.682720968628,0.,34.3094577320604));
#84933=CARTESIAN_POINT('Ctrl Pts',(480.682720968628,-34.3094577320603,34.3094577320603));
#84934=CARTESIAN_POINT('Ctrl Pts',(480.682720968628,-34.3094577320604,0.));
#84935=CARTESIAN_POINT('Ctrl Pts',(480.682720968628,-34.3094577320603,-34.3094577320603));
#84936=CARTESIAN_POINT('Ctrl Pts',(480.682720968628,0.,-34.3094577320604));
#84937=CARTESIAN_POINT('Ctrl Pts',(480.682720968628,34.3094577320603,-34.3094577320603));
#84938=CARTESIAN_POINT('Ctrl Pts',(480.682720968628,34.3094577320604,0.));
#84939=CARTESIAN_POINT('Ctrl Pts',(480.086198305556,33.1532218206079,0.));
#84940=CARTESIAN_POINT('Ctrl Pts',(480.086198305556,33.1532218206079,33.1532218206079));
#84941=CARTESIAN_POINT('Ctrl Pts',(480.086198305556,0.,33.1532218206079));
#84942=CARTESIAN_POINT('Ctrl Pts',(480.086198305556,-33.1532218206079,33.1532218206079));
#84943=CARTESIAN_POINT('Ctrl Pts',(480.086198305556,-33.1532218206079,0.));
#84944=CARTESIAN_POINT('Ctrl Pts',(480.086198305556,-33.1532218206079,-33.1532218206079));
#84945=CARTESIAN_POINT('Ctrl Pts',(480.086198305556,0.,-33.1532218206079));
#84946=CARTESIAN_POINT('Ctrl Pts',(480.086198305556,33.1532218206079,-33.1532218206079));
#84947=CARTESIAN_POINT('Ctrl Pts',(480.086198305556,33.1532218206079,0.));
#84948=CARTESIAN_POINT('Ctrl Pts',(479.480404754155,32.0713081103475,0.));
#84949=CARTESIAN_POINT('Ctrl Pts',(479.480404754155,32.0713081103475,32.0713081103475));
#84950=CARTESIAN_POINT('Ctrl Pts',(479.480404754155,0.,32.0713081103475));
#84951=CARTESIAN_POINT('Ctrl Pts',(479.480404754155,-32.0713081103475,32.0713081103475));
#84952=CARTESIAN_POINT('Ctrl Pts',(479.480404754155,-32.0713081103475,0.));
#84953=CARTESIAN_POINT('Ctrl Pts',(479.480404754155,-32.0713081103475,-32.0713081103475));
#84954=CARTESIAN_POINT('Ctrl Pts',(479.480404754155,0.,-32.0713081103475));
#84955=CARTESIAN_POINT('Ctrl Pts',(479.480404754155,32.0713081103475,-32.0713081103475));
#84956=CARTESIAN_POINT('Ctrl Pts',(479.480404754155,32.0713081103475,0.));
#84957=CARTESIAN_POINT('Ctrl Pts',(478.845896061198,31.1648170165913,0.));
#84958=CARTESIAN_POINT('Ctrl Pts',(478.845896061198,31.1648170165913,31.1648170165913));
#84959=CARTESIAN_POINT('Ctrl Pts',(478.845896061198,0.,31.1648170165913));
#84960=CARTESIAN_POINT('Ctrl Pts',(478.845896061198,-31.1648170165913,31.1648170165913));
#84961=CARTESIAN_POINT('Ctrl Pts',(478.845896061198,-31.1648170165913,0.));
#84962=CARTESIAN_POINT('Ctrl Pts',(478.845896061198,-31.1648170165913,-31.1648170165913));
#84963=CARTESIAN_POINT('Ctrl Pts',(478.845896061198,0.,-31.1648170165913));
#84964=CARTESIAN_POINT('Ctrl Pts',(478.845896061198,31.1648170165913,-31.1648170165913));
#84965=CARTESIAN_POINT('Ctrl Pts',(478.845896061198,31.1648170165913,0.));
#84966=CARTESIAN_POINT('Ctrl Pts',(478.170705434033,30.5212549544916,0.));
#84967=CARTESIAN_POINT('Ctrl Pts',(478.170705434033,30.5212549544916,30.5212549544916));
#84968=CARTESIAN_POINT('Ctrl Pts',(478.170705434033,0.,30.5212549544916));
#84969=CARTESIAN_POINT('Ctrl Pts',(478.170705434033,-30.5212549544916,30.5212549544916));
#84970=CARTESIAN_POINT('Ctrl Pts',(478.170705434033,-30.5212549544916,0.));
#84971=CARTESIAN_POINT('Ctrl Pts',(478.170705434033,-30.5212549544916,-30.5212549544916));
#84972=CARTESIAN_POINT('Ctrl Pts',(478.170705434033,0.,-30.5212549544916));
#84973=CARTESIAN_POINT('Ctrl Pts',(478.170705434033,30.5212549544916,-30.5212549544916));
#84974=CARTESIAN_POINT('Ctrl Pts',(478.170705434033,30.5212549544916,0.));
#84975=CARTESIAN_POINT('Ctrl Pts',(477.454558588677,30.2006533599419,0.));
#84976=CARTESIAN_POINT('Ctrl Pts',(477.454558588677,30.2006533599418,30.2006533599418));
#84977=CARTESIAN_POINT('Ctrl Pts',(477.454558588677,0.,30.2006533599419));
#84978=CARTESIAN_POINT('Ctrl Pts',(477.454558588677,-30.2006533599418,30.2006533599418));
#84979=CARTESIAN_POINT('Ctrl Pts',(477.454558588677,-30.2006533599419,0.));
#84980=CARTESIAN_POINT('Ctrl Pts',(477.454558588677,-30.2006533599418,-30.2006533599418));
#84981=CARTESIAN_POINT('Ctrl Pts',(477.454558588677,0.,-30.2006533599419));
#84982=CARTESIAN_POINT('Ctrl Pts',(477.454558588677,30.2006533599418,-30.2006533599418));
#84983=CARTESIAN_POINT('Ctrl Pts',(477.454558588677,30.2006533599419,0.));
#84984=CARTESIAN_POINT('Ctrl Pts',(476.715088006725,30.2182781872629,0.));
#84985=CARTESIAN_POINT('Ctrl Pts',(476.715088006725,30.2182781872629,30.2182781872629));
#84986=CARTESIAN_POINT('Ctrl Pts',(476.715088006725,0.,30.2182781872629));
#84987=CARTESIAN_POINT('Ctrl Pts',(476.715088006725,-30.2182781872629,30.2182781872629));
#84988=CARTESIAN_POINT('Ctrl Pts',(476.715088006725,-30.2182781872629,0.));
#84989=CARTESIAN_POINT('Ctrl Pts',(476.715088006725,-30.2182781872629,-30.2182781872629));
#84990=CARTESIAN_POINT('Ctrl Pts',(476.715088006725,0.,-30.2182781872629));
#84991=CARTESIAN_POINT('Ctrl Pts',(476.715088006725,30.2182781872629,-30.2182781872629));
#84992=CARTESIAN_POINT('Ctrl Pts',(476.715088006725,30.2182781872629,0.));
#84993=CARTESIAN_POINT('Ctrl Pts',(475.981110865709,30.5489260877444,0.));
#84994=CARTESIAN_POINT('Ctrl Pts',(475.981110865709,30.5489260877443,30.5489260877443));
#84995=CARTESIAN_POINT('Ctrl Pts',(475.981110865709,0.,30.5489260877444));
#84996=CARTESIAN_POINT('Ctrl Pts',(475.981110865709,-30.5489260877443,30.5489260877443));
#84997=CARTESIAN_POINT('Ctrl Pts',(475.981110865709,-30.5489260877444,0.));
#84998=CARTESIAN_POINT('Ctrl Pts',(475.981110865709,-30.5489260877443,-30.5489260877443));
#84999=CARTESIAN_POINT('Ctrl Pts',(475.981110865709,0.,-30.5489260877444));
#85000=CARTESIAN_POINT('Ctrl Pts',(475.981110865709,30.5489260877443,-30.5489260877443));
#85001=CARTESIAN_POINT('Ctrl Pts',(475.981110865709,30.5489260877444,0.));
#85002=CARTESIAN_POINT('Ctrl Pts',(475.281638153934,31.1373046376156,0.));
#85003=CARTESIAN_POINT('Ctrl Pts',(475.281638153934,31.1373046376156,31.1373046376156));
#85004=CARTESIAN_POINT('Ctrl Pts',(475.281638153934,0.,31.1373046376156));
#85005=CARTESIAN_POINT('Ctrl Pts',(475.281638153934,-31.1373046376156,31.1373046376156));
#85006=CARTESIAN_POINT('Ctrl Pts',(475.281638153934,-31.1373046376156,0.));
#85007=CARTESIAN_POINT('Ctrl Pts',(475.281638153934,-31.1373046376156,-31.1373046376156));
#85008=CARTESIAN_POINT('Ctrl Pts',(475.281638153934,0.,-31.1373046376156));
#85009=CARTESIAN_POINT('Ctrl Pts',(475.281638153934,31.1373046376156,-31.1373046376156));
#85010=CARTESIAN_POINT('Ctrl Pts',(475.281638153934,31.1373046376156,0.));
#85011=CARTESIAN_POINT('Ctrl Pts',(474.637420315231,31.9063742772383,0.));
#85012=CARTESIAN_POINT('Ctrl Pts',(474.637420315231,31.9063742772383,31.9063742772383));
#85013=CARTESIAN_POINT('Ctrl Pts',(474.637420315231,0.,31.9063742772383));
#85014=CARTESIAN_POINT('Ctrl Pts',(474.637420315231,-31.9063742772383,31.9063742772383));
#85015=CARTESIAN_POINT('Ctrl Pts',(474.637420315231,-31.9063742772383,0.));
#85016=CARTESIAN_POINT('Ctrl Pts',(474.637420315231,-31.9063742772383,-31.9063742772383));
#85017=CARTESIAN_POINT('Ctrl Pts',(474.637420315231,0.,-31.9063742772383));
#85018=CARTESIAN_POINT('Ctrl Pts',(474.637420315231,31.9063742772383,-31.9063742772383));
#85019=CARTESIAN_POINT('Ctrl Pts',(474.637420315231,31.9063742772383,0.));
#85020=CARTESIAN_POINT('Ctrl Pts',(474.048807350844,32.7664588883108,0.));
#85021=CARTESIAN_POINT('Ctrl Pts',(474.048807350844,32.7664588883108,32.7664588883108));
#85022=CARTESIAN_POINT('Ctrl Pts',(474.048807350844,0.,32.7664588883108));
#85023=CARTESIAN_POINT('Ctrl Pts',(474.048807350844,-32.7664588883108,32.7664588883108));
#85024=CARTESIAN_POINT('Ctrl Pts',(474.048807350844,-32.7664588883108,0.));
#85025=CARTESIAN_POINT('Ctrl Pts',(474.048807350844,-32.7664588883108,-32.7664588883108));
#85026=CARTESIAN_POINT('Ctrl Pts',(474.048807350844,0.,-32.7664588883108));
#85027=CARTESIAN_POINT('Ctrl Pts',(474.048807350844,32.7664588883108,-32.7664588883108));
#85028=CARTESIAN_POINT('Ctrl Pts',(474.048807350844,32.7664588883108,0.));
#85029=CARTESIAN_POINT('Ctrl Pts',(473.496207150892,33.6242325832595,0.));
#85030=CARTESIAN_POINT('Ctrl Pts',(473.496207150892,33.6242325832595,33.6242325832595));
#85031=CARTESIAN_POINT('Ctrl Pts',(473.496207150892,0.,33.6242325832595));
#85032=CARTESIAN_POINT('Ctrl Pts',(473.496207150892,-33.6242325832595,33.6242325832595));
#85033=CARTESIAN_POINT('Ctrl Pts',(473.496207150892,-33.6242325832595,0.));
#85034=CARTESIAN_POINT('Ctrl Pts',(473.496207150892,-33.6242325832595,-33.6242325832595));
#85035=CARTESIAN_POINT('Ctrl Pts',(473.496207150892,0.,-33.6242325832595));
#85036=CARTESIAN_POINT('Ctrl Pts',(473.496207150892,33.6242325832595,-33.6242325832595));
#85037=CARTESIAN_POINT('Ctrl Pts',(473.496207150892,33.6242325832595,0.));
#85038=CARTESIAN_POINT('Ctrl Pts',(472.950173506317,34.3917148430238,0.));
#85039=CARTESIAN_POINT('Ctrl Pts',(472.950173506317,34.3917148430237,34.3917148430237));
#85040=CARTESIAN_POINT('Ctrl Pts',(472.950173506317,0.,34.3917148430238));
#85041=CARTESIAN_POINT('Ctrl Pts',(472.950173506317,-34.3917148430237,34.3917148430237));
#85042=CARTESIAN_POINT('Ctrl Pts',(472.950173506317,-34.3917148430238,0.));
#85043=CARTESIAN_POINT('Ctrl Pts',(472.950173506317,-34.3917148430237,-34.3917148430237));
#85044=CARTESIAN_POINT('Ctrl Pts',(472.950173506317,0.,-34.3917148430238));
#85045=CARTESIAN_POINT('Ctrl Pts',(472.950173506317,34.3917148430237,-34.3917148430237));
#85046=CARTESIAN_POINT('Ctrl Pts',(472.950173506317,34.3917148430238,0.));
#85047=CARTESIAN_POINT('Ctrl Pts',(472.379062231055,34.9957749951357,0.));
#85048=CARTESIAN_POINT('Ctrl Pts',(472.379062231055,34.9957749951357,34.9957749951357));
#85049=CARTESIAN_POINT('Ctrl Pts',(472.379062231055,0.,34.9957749951357));
#85050=CARTESIAN_POINT('Ctrl Pts',(472.379062231055,-34.9957749951357,34.9957749951357));
#85051=CARTESIAN_POINT('Ctrl Pts',(472.379062231055,-34.9957749951357,0.));
#85052=CARTESIAN_POINT('Ctrl Pts',(472.379062231055,-34.9957749951357,-34.9957749951357));
#85053=CARTESIAN_POINT('Ctrl Pts',(472.379062231055,0.,-34.9957749951357));
#85054=CARTESIAN_POINT('Ctrl Pts',(472.379062231055,34.9957749951357,-34.9957749951357));
#85055=CARTESIAN_POINT('Ctrl Pts',(472.379062231055,34.9957749951357,0.));
#85056=CARTESIAN_POINT('Ctrl Pts',(471.756985572081,35.3862684299237,0.));
#85057=CARTESIAN_POINT('Ctrl Pts',(471.756985572081,35.3862684299237,35.3862684299237));
#85058=CARTESIAN_POINT('Ctrl Pts',(471.756985572081,0.,35.3862684299237));
#85059=CARTESIAN_POINT('Ctrl Pts',(471.756985572081,-35.3862684299237,35.3862684299237));
#85060=CARTESIAN_POINT('Ctrl Pts',(471.756985572081,-35.3862684299237,0.));
#85061=CARTESIAN_POINT('Ctrl Pts',(471.756985572081,-35.3862684299237,-35.3862684299237));
#85062=CARTESIAN_POINT('Ctrl Pts',(471.756985572081,0.,-35.3862684299237));
#85063=CARTESIAN_POINT('Ctrl Pts',(471.756985572081,35.3862684299237,-35.3862684299237));
#85064=CARTESIAN_POINT('Ctrl Pts',(471.756985572081,35.3862684299237,0.));
#85065=CARTESIAN_POINT('Ctrl Pts',(471.073330047455,35.547602310438,0.));
#85066=CARTESIAN_POINT('Ctrl Pts',(471.073330047455,35.547602310438,35.547602310438));
#85067=CARTESIAN_POINT('Ctrl Pts',(471.073330047455,0.,35.547602310438));
#85068=CARTESIAN_POINT('Ctrl Pts',(471.073330047455,-35.547602310438,35.547602310438));
#85069=CARTESIAN_POINT('Ctrl Pts',(471.073330047455,-35.547602310438,0.));
#85070=CARTESIAN_POINT('Ctrl Pts',(471.073330047455,-35.547602310438,-35.547602310438));
#85071=CARTESIAN_POINT('Ctrl Pts',(471.073330047455,0.,-35.547602310438));
#85072=CARTESIAN_POINT('Ctrl Pts',(471.073330047455,35.547602310438,-35.547602310438));
#85073=CARTESIAN_POINT('Ctrl Pts',(471.073330047455,35.547602310438,0.));
#85074=CARTESIAN_POINT('Ctrl Pts',(470.335597351742,35.4987206841576,0.));
#85075=CARTESIAN_POINT('Ctrl Pts',(470.335597351742,35.4987206841576,35.4987206841576));
#85076=CARTESIAN_POINT('Ctrl Pts',(470.335597351742,0.,35.4987206841576));
#85077=CARTESIAN_POINT('Ctrl Pts',(470.335597351742,-35.4987206841576,35.4987206841576));
#85078=CARTESIAN_POINT('Ctrl Pts',(470.335597351742,-35.4987206841576,0.));
#85079=CARTESIAN_POINT('Ctrl Pts',(470.335597351742,-35.4987206841576,-35.4987206841576));
#85080=CARTESIAN_POINT('Ctrl Pts',(470.335597351742,0.,-35.4987206841576));
#85081=CARTESIAN_POINT('Ctrl Pts',(470.335597351742,35.4987206841576,-35.4987206841576));
#85082=CARTESIAN_POINT('Ctrl Pts',(470.335597351742,35.4987206841576,0.));
#85083=CARTESIAN_POINT('Ctrl Pts',(469.561546477286,35.2747783728489,0.));
#85084=CARTESIAN_POINT('Ctrl Pts',(469.561546477286,35.2747783728489,35.2747783728489));
#85085=CARTESIAN_POINT('Ctrl Pts',(469.561546477286,0.,35.2747783728489));
#85086=CARTESIAN_POINT('Ctrl Pts',(469.561546477286,-35.2747783728489,35.2747783728489));
#85087=CARTESIAN_POINT('Ctrl Pts',(469.561546477286,-35.2747783728489,0.));
#85088=CARTESIAN_POINT('Ctrl Pts',(469.561546477286,-35.2747783728489,-35.2747783728489));
#85089=CARTESIAN_POINT('Ctrl Pts',(469.561546477286,0.,-35.2747783728489));
#85090=CARTESIAN_POINT('Ctrl Pts',(469.561546477286,35.2747783728489,-35.2747783728489));
#85091=CARTESIAN_POINT('Ctrl Pts',(469.561546477286,35.2747783728489,0.));
#85092=CARTESIAN_POINT('Ctrl Pts',(468.774141019888,34.9141595380048,0.));
#85093=CARTESIAN_POINT('Ctrl Pts',(468.774141019888,34.9141595380048,34.9141595380048));
#85094=CARTESIAN_POINT('Ctrl Pts',(468.774141019888,0.,34.9141595380048));
#85095=CARTESIAN_POINT('Ctrl Pts',(468.774141019888,-34.9141595380048,34.9141595380048));
#85096=CARTESIAN_POINT('Ctrl Pts',(468.774141019888,-34.9141595380048,0.));
#85097=CARTESIAN_POINT('Ctrl Pts',(468.774141019888,-34.9141595380048,-34.9141595380048));
#85098=CARTESIAN_POINT('Ctrl Pts',(468.774141019888,0.,-34.9141595380048));
#85099=CARTESIAN_POINT('Ctrl Pts',(468.774141019888,34.9141595380048,-34.9141595380048));
#85100=CARTESIAN_POINT('Ctrl Pts',(468.774141019888,34.9141595380048,0.));
#85101=CARTESIAN_POINT('Ctrl Pts',(467.994839856681,34.4411672254374,0.));
#85102=CARTESIAN_POINT('Ctrl Pts',(467.994839856681,34.4411672254374,34.4411672254374));
#85103=CARTESIAN_POINT('Ctrl Pts',(467.994839856681,0.,34.4411672254374));
#85104=CARTESIAN_POINT('Ctrl Pts',(467.994839856681,-34.4411672254374,34.4411672254374));
#85105=CARTESIAN_POINT('Ctrl Pts',(467.994839856681,-34.4411672254374,0.));
#85106=CARTESIAN_POINT('Ctrl Pts',(467.994839856681,-34.4411672254374,-34.4411672254374));
#85107=CARTESIAN_POINT('Ctrl Pts',(467.994839856681,0.,-34.4411672254374));
#85108=CARTESIAN_POINT('Ctrl Pts',(467.994839856681,34.4411672254374,-34.4411672254374));
#85109=CARTESIAN_POINT('Ctrl Pts',(467.994839856681,34.4411672254374,0.));
#85110=CARTESIAN_POINT('Ctrl Pts',(467.239271643519,33.8574930279435,0.));
#85111=CARTESIAN_POINT('Ctrl Pts',(467.239271643519,33.8574930279435,33.8574930279435));
#85112=CARTESIAN_POINT('Ctrl Pts',(467.239271643519,0.,33.8574930279435));
#85113=CARTESIAN_POINT('Ctrl Pts',(467.239271643519,-33.8574930279435,33.8574930279435));
#85114=CARTESIAN_POINT('Ctrl Pts',(467.239271643519,-33.8574930279435,0.));
#85115=CARTESIAN_POINT('Ctrl Pts',(467.239271643519,-33.8574930279435,-33.8574930279435));
#85116=CARTESIAN_POINT('Ctrl Pts',(467.239271643519,0.,-33.8574930279435));
#85117=CARTESIAN_POINT('Ctrl Pts',(467.239271643519,33.8574930279435,-33.8574930279435));
#85118=CARTESIAN_POINT('Ctrl Pts',(467.239271643519,33.8574930279435,0.));
#85119=CARTESIAN_POINT('Ctrl Pts',(466.517752610425,33.1545694480525,0.));
#85120=CARTESIAN_POINT('Ctrl Pts',(466.517752610425,33.1545694480525,33.1545694480525));
#85121=CARTESIAN_POINT('Ctrl Pts',(466.517752610425,0.,33.1545694480525));
#85122=CARTESIAN_POINT('Ctrl Pts',(466.517752610425,-33.1545694480525,33.1545694480525));
#85123=CARTESIAN_POINT('Ctrl Pts',(466.517752610425,-33.1545694480525,0.));
#85124=CARTESIAN_POINT('Ctrl Pts',(466.517752610425,-33.1545694480525,-33.1545694480525));
#85125=CARTESIAN_POINT('Ctrl Pts',(466.517752610425,0.,-33.1545694480525));
#85126=CARTESIAN_POINT('Ctrl Pts',(466.517752610425,33.1545694480525,-33.1545694480525));
#85127=CARTESIAN_POINT('Ctrl Pts',(466.517752610425,33.1545694480525,0.));
#85128=CARTESIAN_POINT('Ctrl Pts',(465.834971562565,32.3218329216103,0.));
#85129=CARTESIAN_POINT('Ctrl Pts',(465.834971562565,32.3218329216103,32.3218329216103));
#85130=CARTESIAN_POINT('Ctrl Pts',(465.834971562565,0.,32.3218329216103));
#85131=CARTESIAN_POINT('Ctrl Pts',(465.834971562565,-32.3218329216103,32.3218329216103));
#85132=CARTESIAN_POINT('Ctrl Pts',(465.834971562565,-32.3218329216103,0.));
#85133=CARTESIAN_POINT('Ctrl Pts',(465.834971562565,-32.3218329216103,-32.3218329216103));
#85134=CARTESIAN_POINT('Ctrl Pts',(465.834971562565,0.,-32.3218329216103));
#85135=CARTESIAN_POINT('Ctrl Pts',(465.834971562565,32.3218329216103,-32.3218329216103));
#85136=CARTESIAN_POINT('Ctrl Pts',(465.834971562565,32.3218329216103,0.));
#85137=CARTESIAN_POINT('Ctrl Pts',(465.189920345436,31.3570687154993,0.));
#85138=CARTESIAN_POINT('Ctrl Pts',(465.189920345436,31.3570687154992,31.3570687154992));
#85139=CARTESIAN_POINT('Ctrl Pts',(465.189920345436,0.,31.3570687154993));
#85140=CARTESIAN_POINT('Ctrl Pts',(465.189920345436,-31.3570687154992,31.3570687154992));
#85141=CARTESIAN_POINT('Ctrl Pts',(465.189920345436,-31.3570687154993,0.));
#85142=CARTESIAN_POINT('Ctrl Pts',(465.189920345436,-31.3570687154992,-31.3570687154992));
#85143=CARTESIAN_POINT('Ctrl Pts',(465.189920345436,0.,-31.3570687154993));
#85144=CARTESIAN_POINT('Ctrl Pts',(465.189920345436,31.3570687154992,-31.3570687154992));
#85145=CARTESIAN_POINT('Ctrl Pts',(465.189920345436,31.3570687154993,0.));
#85146=CARTESIAN_POINT('Ctrl Pts',(464.575897029354,30.2747905161882,0.));
#85147=CARTESIAN_POINT('Ctrl Pts',(464.575897029354,30.2747905161882,30.2747905161882));
#85148=CARTESIAN_POINT('Ctrl Pts',(464.575897029354,0.,30.2747905161882));
#85149=CARTESIAN_POINT('Ctrl Pts',(464.575897029354,-30.2747905161882,30.2747905161882));
#85150=CARTESIAN_POINT('Ctrl Pts',(464.575897029354,-30.2747905161882,0.));
#85151=CARTESIAN_POINT('Ctrl Pts',(464.575897029354,-30.2747905161882,-30.2747905161882));
#85152=CARTESIAN_POINT('Ctrl Pts',(464.575897029354,0.,-30.2747905161882));
#85153=CARTESIAN_POINT('Ctrl Pts',(464.575897029354,30.2747905161882,-30.2747905161882));
#85154=CARTESIAN_POINT('Ctrl Pts',(464.575897029354,30.2747905161882,0.));
#85155=CARTESIAN_POINT('Ctrl Pts',(463.980012926408,29.1182237614132,0.));
#85156=CARTESIAN_POINT('Ctrl Pts',(463.980012926408,29.1182237614132,29.1182237614132));
#85157=CARTESIAN_POINT('Ctrl Pts',(463.980012926408,0.,29.1182237614132));
#85158=CARTESIAN_POINT('Ctrl Pts',(463.980012926408,-29.1182237614132,29.1182237614132));
#85159=CARTESIAN_POINT('Ctrl Pts',(463.980012926408,-29.1182237614132,0.));
#85160=CARTESIAN_POINT('Ctrl Pts',(463.980012926408,-29.1182237614132,-29.1182237614132));
#85161=CARTESIAN_POINT('Ctrl Pts',(463.980012926408,0.,-29.1182237614132));
#85162=CARTESIAN_POINT('Ctrl Pts',(463.980012926408,29.1182237614132,-29.1182237614132));
#85163=CARTESIAN_POINT('Ctrl Pts',(463.980012926408,29.1182237614132,0.));
#85164=CARTESIAN_POINT('Ctrl Pts',(463.38544807492,27.9547399267918,0.));
#85165=CARTESIAN_POINT('Ctrl Pts',(463.38544807492,27.9547399267918,27.9547399267918));
#85166=CARTESIAN_POINT('Ctrl Pts',(463.38544807492,0.,27.9547399267918));
#85167=CARTESIAN_POINT('Ctrl Pts',(463.38544807492,-27.9547399267918,27.9547399267918));
#85168=CARTESIAN_POINT('Ctrl Pts',(463.38544807492,-27.9547399267918,0.));
#85169=CARTESIAN_POINT('Ctrl Pts',(463.38544807492,-27.9547399267918,-27.9547399267918));
#85170=CARTESIAN_POINT('Ctrl Pts',(463.38544807492,0.,-27.9547399267918));
#85171=CARTESIAN_POINT('Ctrl Pts',(463.38544807492,27.9547399267918,-27.9547399267918));
#85172=CARTESIAN_POINT('Ctrl Pts',(463.38544807492,27.9547399267918,0.));
#85173=CARTESIAN_POINT('Ctrl Pts',(462.775015619175,26.8639618331474,0.));
#85174=CARTESIAN_POINT('Ctrl Pts',(462.775015619175,26.8639618331474,26.8639618331474));
#85175=CARTESIAN_POINT('Ctrl Pts',(462.775015619175,0.,26.8639618331474));
#85176=CARTESIAN_POINT('Ctrl Pts',(462.775015619175,-26.8639618331474,26.8639618331474));
#85177=CARTESIAN_POINT('Ctrl Pts',(462.775015619175,-26.8639618331474,0.));
#85178=CARTESIAN_POINT('Ctrl Pts',(462.775015619175,-26.8639618331474,-26.8639618331474));
#85179=CARTESIAN_POINT('Ctrl Pts',(462.775015619175,0.,-26.8639618331474));
#85180=CARTESIAN_POINT('Ctrl Pts',(462.775015619175,26.8639618331474,-26.8639618331474));
#85181=CARTESIAN_POINT('Ctrl Pts',(462.775015619175,26.8639618331474,0.));
#85182=CARTESIAN_POINT('Ctrl Pts',(462.134199633467,25.9283453171447,0.));
#85183=CARTESIAN_POINT('Ctrl Pts',(462.134199633467,25.9283453171447,25.9283453171447));
#85184=CARTESIAN_POINT('Ctrl Pts',(462.134199633467,0.,25.9283453171447));
#85185=CARTESIAN_POINT('Ctrl Pts',(462.134199633467,-25.9283453171447,25.9283453171447));
#85186=CARTESIAN_POINT('Ctrl Pts',(462.134199633467,-25.9283453171447,0.));
#85187=CARTESIAN_POINT('Ctrl Pts',(462.134199633467,-25.9283453171447,-25.9283453171447));
#85188=CARTESIAN_POINT('Ctrl Pts',(462.134199633467,0.,-25.9283453171447));
#85189=CARTESIAN_POINT('Ctrl Pts',(462.134199633467,25.9283453171447,-25.9283453171447));
#85190=CARTESIAN_POINT('Ctrl Pts',(462.134199633467,25.9283453171447,0.));
#85191=CARTESIAN_POINT('Ctrl Pts',(461.454649264338,25.2224382685937,0.));
#85192=CARTESIAN_POINT('Ctrl Pts',(461.454649264338,25.2224382685937,25.2224382685937));
#85193=CARTESIAN_POINT('Ctrl Pts',(461.454649264338,0.,25.2224382685937));
#85194=CARTESIAN_POINT('Ctrl Pts',(461.454649264338,-25.2224382685937,25.2224382685937));
#85195=CARTESIAN_POINT('Ctrl Pts',(461.454649264338,-25.2224382685937,0.));
#85196=CARTESIAN_POINT('Ctrl Pts',(461.454649264338,-25.2224382685937,-25.2224382685937));
#85197=CARTESIAN_POINT('Ctrl Pts',(461.454649264338,0.,-25.2224382685937));
#85198=CARTESIAN_POINT('Ctrl Pts',(461.454649264338,25.2224382685937,-25.2224382685937));
#85199=CARTESIAN_POINT('Ctrl Pts',(461.454649264338,25.2224382685937,0.));
#85200=CARTESIAN_POINT('Ctrl Pts',(460.736933199464,24.8033903723626,0.));
#85201=CARTESIAN_POINT('Ctrl Pts',(460.736933199464,24.8033903723626,24.8033903723626));
#85202=CARTESIAN_POINT('Ctrl Pts',(460.736933199464,0.,24.8033903723626));
#85203=CARTESIAN_POINT('Ctrl Pts',(460.736933199464,-24.8033903723626,24.8033903723626));
#85204=CARTESIAN_POINT('Ctrl Pts',(460.736933199464,-24.8033903723626,0.));
#85205=CARTESIAN_POINT('Ctrl Pts',(460.736933199464,-24.8033903723626,-24.8033903723626));
#85206=CARTESIAN_POINT('Ctrl Pts',(460.736933199464,0.,-24.8033903723626));
#85207=CARTESIAN_POINT('Ctrl Pts',(460.736933199464,24.8033903723626,-24.8033903723626));
#85208=CARTESIAN_POINT('Ctrl Pts',(460.736933199464,24.8033903723626,0.));
#85209=CARTESIAN_POINT('Ctrl Pts',(459.994949810424,24.6992460116247,0.));
#85210=CARTESIAN_POINT('Ctrl Pts',(459.994949810424,24.6992460116247,24.6992460116247));
#85211=CARTESIAN_POINT('Ctrl Pts',(459.994949810424,0.,24.6992460116247));
#85212=CARTESIAN_POINT('Ctrl Pts',(459.994949810424,-24.6992460116247,24.6992460116247));
#85213=CARTESIAN_POINT('Ctrl Pts',(459.994949810424,-24.6992460116247,0.));
#85214=CARTESIAN_POINT('Ctrl Pts',(459.994949810424,-24.6992460116247,-24.6992460116247));
#85215=CARTESIAN_POINT('Ctrl Pts',(459.994949810424,0.,-24.6992460116247));
#85216=CARTESIAN_POINT('Ctrl Pts',(459.994949810424,24.6992460116247,-24.6992460116247));
#85217=CARTESIAN_POINT('Ctrl Pts',(459.994949810424,24.6992460116247,0.));
#85218=CARTESIAN_POINT('Ctrl Pts',(459.255007342274,24.9039206717732,0.));
#85219=CARTESIAN_POINT('Ctrl Pts',(459.255007342274,24.9039206717732,24.9039206717732));
#85220=CARTESIAN_POINT('Ctrl Pts',(459.255007342274,0.,24.9039206717732));
#85221=CARTESIAN_POINT('Ctrl Pts',(459.255007342274,-24.9039206717732,24.9039206717732));
#85222=CARTESIAN_POINT('Ctrl Pts',(459.255007342274,-24.9039206717732,0.));
#85223=CARTESIAN_POINT('Ctrl Pts',(459.255007342274,-24.9039206717732,-24.9039206717732));
#85224=CARTESIAN_POINT('Ctrl Pts',(459.255007342274,0.,-24.9039206717732));
#85225=CARTESIAN_POINT('Ctrl Pts',(459.255007342274,24.9039206717732,-24.9039206717732));
#85226=CARTESIAN_POINT('Ctrl Pts',(459.255007342274,24.9039206717732,0.));
#85227=CARTESIAN_POINT('Ctrl Pts',(458.545378831534,25.3834939706622,0.));
#85228=CARTESIAN_POINT('Ctrl Pts',(458.545378831534,25.3834939706622,25.3834939706622));
#85229=CARTESIAN_POINT('Ctrl Pts',(458.545378831534,0.,25.3834939706622));
#85230=CARTESIAN_POINT('Ctrl Pts',(458.545378831534,-25.3834939706622,25.3834939706622));
#85231=CARTESIAN_POINT('Ctrl Pts',(458.545378831534,-25.3834939706622,0.));
#85232=CARTESIAN_POINT('Ctrl Pts',(458.545378831534,-25.3834939706622,-25.3834939706622));
#85233=CARTESIAN_POINT('Ctrl Pts',(458.545378831534,0.,-25.3834939706622));
#85234=CARTESIAN_POINT('Ctrl Pts',(458.545378831534,25.3834939706622,-25.3834939706622));
#85235=CARTESIAN_POINT('Ctrl Pts',(458.545378831534,25.3834939706622,0.));
#85236=CARTESIAN_POINT('Ctrl Pts',(457.888379201951,26.0800747021197,0.));
#85237=CARTESIAN_POINT('Ctrl Pts',(457.888379201951,26.0800747021197,26.0800747021197));
#85238=CARTESIAN_POINT('Ctrl Pts',(457.888379201951,0.,26.0800747021197));
#85239=CARTESIAN_POINT('Ctrl Pts',(457.888379201951,-26.0800747021197,26.0800747021197));
#85240=CARTESIAN_POINT('Ctrl Pts',(457.888379201951,-26.0800747021197,0.));
#85241=CARTESIAN_POINT('Ctrl Pts',(457.888379201951,-26.0800747021197,-26.0800747021197));
#85242=CARTESIAN_POINT('Ctrl Pts',(457.888379201951,0.,-26.0800747021197));
#85243=CARTESIAN_POINT('Ctrl Pts',(457.888379201951,26.0800747021197,-26.0800747021197));
#85244=CARTESIAN_POINT('Ctrl Pts',(457.888379201951,26.0800747021197,0.));
#85245=CARTESIAN_POINT('Ctrl Pts',(457.290615845749,26.9163263890247,0.));
#85246=CARTESIAN_POINT('Ctrl Pts',(457.290615845749,26.9163263890247,26.9163263890247));
#85247=CARTESIAN_POINT('Ctrl Pts',(457.290615845749,0.,26.9163263890247));
#85248=CARTESIAN_POINT('Ctrl Pts',(457.290615845749,-26.9163263890247,26.9163263890247));
#85249=CARTESIAN_POINT('Ctrl Pts',(457.290615845749,-26.9163263890247,0.));
#85250=CARTESIAN_POINT('Ctrl Pts',(457.290615845749,-26.9163263890247,-26.9163263890247));
#85251=CARTESIAN_POINT('Ctrl Pts',(457.290615845749,0.,-26.9163263890247));
#85252=CARTESIAN_POINT('Ctrl Pts',(457.290615845749,26.9163263890247,-26.9163263890247));
#85253=CARTESIAN_POINT('Ctrl Pts',(457.290615845749,26.9163263890247,0.));
#85254=CARTESIAN_POINT('Ctrl Pts',(456.736386522373,27.8005738327045,0.));
#85255=CARTESIAN_POINT('Ctrl Pts',(456.736386522373,27.8005738327045,27.8005738327045));
#85256=CARTESIAN_POINT('Ctrl Pts',(456.736386522373,0.,27.8005738327045));
#85257=CARTESIAN_POINT('Ctrl Pts',(456.736386522373,-27.8005738327045,27.8005738327045));
#85258=CARTESIAN_POINT('Ctrl Pts',(456.736386522373,-27.8005738327045,0.));
#85259=CARTESIAN_POINT('Ctrl Pts',(456.736386522373,-27.8005738327045,-27.8005738327045));
#85260=CARTESIAN_POINT('Ctrl Pts',(456.736386522373,0.,-27.8005738327045));
#85261=CARTESIAN_POINT('Ctrl Pts',(456.736386522373,27.8005738327045,-27.8005738327045));
#85262=CARTESIAN_POINT('Ctrl Pts',(456.736386522373,27.8005738327045,0.));
#85263=CARTESIAN_POINT('Ctrl Pts',(456.197496723491,28.6382733820605,0.));
#85264=CARTESIAN_POINT('Ctrl Pts',(456.197496723491,28.6382733820605,28.6382733820605));
#85265=CARTESIAN_POINT('Ctrl Pts',(456.197496723491,0.,28.6382733820605));
#85266=CARTESIAN_POINT('Ctrl Pts',(456.197496723491,-28.6382733820605,28.6382733820605));
#85267=CARTESIAN_POINT('Ctrl Pts',(456.197496723491,-28.6382733820605,0.));
#85268=CARTESIAN_POINT('Ctrl Pts',(456.197496723491,-28.6382733820605,-28.6382733820605));
#85269=CARTESIAN_POINT('Ctrl Pts',(456.197496723491,0.,-28.6382733820605));
#85270=CARTESIAN_POINT('Ctrl Pts',(456.197496723491,28.6382733820605,-28.6382733820605));
#85271=CARTESIAN_POINT('Ctrl Pts',(456.197496723491,28.6382733820605,0.));
#85272=CARTESIAN_POINT('Ctrl Pts',(455.641185904649,29.3426365369257,0.));
#85273=CARTESIAN_POINT('Ctrl Pts',(455.641185904649,29.3426365369257,29.3426365369257));
#85274=CARTESIAN_POINT('Ctrl Pts',(455.641185904649,0.,29.3426365369257));
#85275=CARTESIAN_POINT('Ctrl Pts',(455.641185904649,-29.3426365369257,29.3426365369257));
#85276=CARTESIAN_POINT('Ctrl Pts',(455.641185904649,-29.3426365369257,0.));
#85277=CARTESIAN_POINT('Ctrl Pts',(455.641185904649,-29.3426365369257,-29.3426365369257));
#85278=CARTESIAN_POINT('Ctrl Pts',(455.641185904649,0.,-29.3426365369257));
#85279=CARTESIAN_POINT('Ctrl Pts',(455.641185904649,29.3426365369257,-29.3426365369257));
#85280=CARTESIAN_POINT('Ctrl Pts',(455.641185904649,29.3426365369257,0.));
#85281=CARTESIAN_POINT('Ctrl Pts',(455.038839374707,29.8456839543521,0.));
#85282=CARTESIAN_POINT('Ctrl Pts',(455.038839374707,29.8456839543521,29.8456839543521));
#85283=CARTESIAN_POINT('Ctrl Pts',(455.038839374707,0.,29.8456839543521));
#85284=CARTESIAN_POINT('Ctrl Pts',(455.038839374707,-29.8456839543521,29.8456839543521));
#85285=CARTESIAN_POINT('Ctrl Pts',(455.038839374707,-29.8456839543521,0.));
#85286=CARTESIAN_POINT('Ctrl Pts',(455.038839374707,-29.8456839543521,-29.8456839543521));
#85287=CARTESIAN_POINT('Ctrl Pts',(455.038839374707,0.,-29.8456839543521));
#85288=CARTESIAN_POINT('Ctrl Pts',(455.038839374707,29.8456839543521,-29.8456839543521));
#85289=CARTESIAN_POINT('Ctrl Pts',(455.038839374707,29.8456839543521,0.));
#85290=CARTESIAN_POINT('Ctrl Pts',(454.374221692176,30.1089010904408,0.));
#85291=CARTESIAN_POINT('Ctrl Pts',(454.374221692176,30.1089010904408,30.1089010904408));
#85292=CARTESIAN_POINT('Ctrl Pts',(454.374221692176,0.,30.1089010904408));
#85293=CARTESIAN_POINT('Ctrl Pts',(454.374221692176,-30.1089010904408,30.1089010904408));
#85294=CARTESIAN_POINT('Ctrl Pts',(454.374221692176,-30.1089010904408,0.));
#85295=CARTESIAN_POINT('Ctrl Pts',(454.374221692176,-30.1089010904408,-30.1089010904408));
#85296=CARTESIAN_POINT('Ctrl Pts',(454.374221692176,0.,-30.1089010904408));
#85297=CARTESIAN_POINT('Ctrl Pts',(454.374221692176,30.1089010904408,-30.1089010904408));
#85298=CARTESIAN_POINT('Ctrl Pts',(454.374221692176,30.1089010904408,0.));
#85299=CARTESIAN_POINT('Ctrl Pts',(453.65232362069,30.1347085607613,0.));
#85300=CARTESIAN_POINT('Ctrl Pts',(453.65232362069,30.1347085607613,30.1347085607613));
#85301=CARTESIAN_POINT('Ctrl Pts',(453.65232362069,0.,30.1347085607613));
#85302=CARTESIAN_POINT('Ctrl Pts',(453.65232362069,-30.1347085607613,30.1347085607613));
#85303=CARTESIAN_POINT('Ctrl Pts',(453.65232362069,-30.1347085607613,0.));
#85304=CARTESIAN_POINT('Ctrl Pts',(453.65232362069,-30.1347085607613,-30.1347085607613));
#85305=CARTESIAN_POINT('Ctrl Pts',(453.65232362069,0.,-30.1347085607613));
#85306=CARTESIAN_POINT('Ctrl Pts',(453.65232362069,30.1347085607613,-30.1347085607613));
#85307=CARTESIAN_POINT('Ctrl Pts',(453.65232362069,30.1347085607613,0.));
#85308=CARTESIAN_POINT('Ctrl Pts',(452.892185119924,29.9520957467627,0.));
#85309=CARTESIAN_POINT('Ctrl Pts',(452.892185119924,29.9520957467627,29.9520957467627));
#85310=CARTESIAN_POINT('Ctrl Pts',(452.892185119924,0.,29.9520957467627));
#85311=CARTESIAN_POINT('Ctrl Pts',(452.892185119924,-29.9520957467627,29.9520957467627));
#85312=CARTESIAN_POINT('Ctrl Pts',(452.892185119924,-29.9520957467627,0.));
#85313=CARTESIAN_POINT('Ctrl Pts',(452.892185119924,-29.9520957467627,-29.9520957467627));
#85314=CARTESIAN_POINT('Ctrl Pts',(452.892185119924,0.,-29.9520957467627));
#85315=CARTESIAN_POINT('Ctrl Pts',(452.892185119924,29.9520957467627,-29.9520957467627));
#85316=CARTESIAN_POINT('Ctrl Pts',(452.892185119924,29.9520957467627,0.));
#85317=CARTESIAN_POINT('Ctrl Pts',(452.119011172215,29.6009203712207,0.));
#85318=CARTESIAN_POINT('Ctrl Pts',(452.119011172215,29.6009203712207,29.6009203712207));
#85319=CARTESIAN_POINT('Ctrl Pts',(452.119011172215,0.,29.6009203712207));
#85320=CARTESIAN_POINT('Ctrl Pts',(452.119011172215,-29.6009203712207,29.6009203712207));
#85321=CARTESIAN_POINT('Ctrl Pts',(452.119011172215,-29.6009203712207,0.));
#85322=CARTESIAN_POINT('Ctrl Pts',(452.119011172215,-29.6009203712207,-29.6009203712207));
#85323=CARTESIAN_POINT('Ctrl Pts',(452.119011172215,0.,-29.6009203712207));
#85324=CARTESIAN_POINT('Ctrl Pts',(452.119011172215,29.6009203712207,-29.6009203712207));
#85325=CARTESIAN_POINT('Ctrl Pts',(452.119011172215,29.6009203712207,0.));
#85326=CARTESIAN_POINT('Ctrl Pts',(451.356904731652,29.117599269821,0.));
#85327=CARTESIAN_POINT('Ctrl Pts',(451.356904731652,29.117599269821,29.117599269821));
#85328=CARTESIAN_POINT('Ctrl Pts',(451.356904731652,0.,29.117599269821));
#85329=CARTESIAN_POINT('Ctrl Pts',(451.356904731652,-29.117599269821,29.117599269821));
#85330=CARTESIAN_POINT('Ctrl Pts',(451.356904731652,-29.117599269821,0.));
#85331=CARTESIAN_POINT('Ctrl Pts',(451.356904731652,-29.117599269821,-29.117599269821));
#85332=CARTESIAN_POINT('Ctrl Pts',(451.356904731652,0.,-29.117599269821));
#85333=CARTESIAN_POINT('Ctrl Pts',(451.356904731652,29.117599269821,-29.117599269821));
#85334=CARTESIAN_POINT('Ctrl Pts',(451.356904731652,29.117599269821,0.));
#85335=CARTESIAN_POINT('Ctrl Pts',(450.6204304333,28.5179209746754,0.));
#85336=CARTESIAN_POINT('Ctrl Pts',(450.6204304333,28.5179209746754,28.5179209746754));
#85337=CARTESIAN_POINT('Ctrl Pts',(450.6204304333,0.,28.5179209746754));
#85338=CARTESIAN_POINT('Ctrl Pts',(450.6204304333,-28.5179209746754,28.5179209746754));
#85339=CARTESIAN_POINT('Ctrl Pts',(450.6204304333,-28.5179209746754,0.));
#85340=CARTESIAN_POINT('Ctrl Pts',(450.6204304333,-28.5179209746754,-28.5179209746754));
#85341=CARTESIAN_POINT('Ctrl Pts',(450.6204304333,0.,-28.5179209746754));
#85342=CARTESIAN_POINT('Ctrl Pts',(450.6204304333,28.5179209746754,-28.5179209746754));
#85343=CARTESIAN_POINT('Ctrl Pts',(450.6204304333,28.5179209746754,0.));
#85344=CARTESIAN_POINT('Ctrl Pts',(449.91530974049,27.8028078305578,0.));
#85345=CARTESIAN_POINT('Ctrl Pts',(449.91530974049,27.8028078305578,27.8028078305578));
#85346=CARTESIAN_POINT('Ctrl Pts',(449.91530974049,0.,27.8028078305578));
#85347=CARTESIAN_POINT('Ctrl Pts',(449.91530974049,-27.8028078305578,27.8028078305578));
#85348=CARTESIAN_POINT('Ctrl Pts',(449.91530974049,-27.8028078305578,0.));
#85349=CARTESIAN_POINT('Ctrl Pts',(449.91530974049,-27.8028078305578,-27.8028078305578));
#85350=CARTESIAN_POINT('Ctrl Pts',(449.91530974049,0.,-27.8028078305578));
#85351=CARTESIAN_POINT('Ctrl Pts',(449.91530974049,27.8028078305578,-27.8028078305578));
#85352=CARTESIAN_POINT('Ctrl Pts',(449.91530974049,27.8028078305578,0.));
#85353=CARTESIAN_POINT('Ctrl Pts',(449.240699204464,26.9680450110966,0.));
#85354=CARTESIAN_POINT('Ctrl Pts',(449.240699204464,26.9680450110966,26.9680450110966));
#85355=CARTESIAN_POINT('Ctrl Pts',(449.240699204464,0.,26.9680450110966));
#85356=CARTESIAN_POINT('Ctrl Pts',(449.240699204464,-26.9680450110966,26.9680450110966));
#85357=CARTESIAN_POINT('Ctrl Pts',(449.240699204464,-26.9680450110966,0.));
#85358=CARTESIAN_POINT('Ctrl Pts',(449.240699204464,-26.9680450110966,-26.9680450110966));
#85359=CARTESIAN_POINT('Ctrl Pts',(449.240699204464,0.,-26.9680450110966));
#85360=CARTESIAN_POINT('Ctrl Pts',(449.240699204464,26.9680450110966,-26.9680450110966));
#85361=CARTESIAN_POINT('Ctrl Pts',(449.240699204464,26.9680450110966,0.));
#85362=CARTESIAN_POINT('Ctrl Pts',(448.590917961239,26.0126948878623,0.));
#85363=CARTESIAN_POINT('Ctrl Pts',(448.590917961239,26.0126948878623,26.0126948878623));
#85364=CARTESIAN_POINT('Ctrl Pts',(448.590917961239,0.,26.0126948878623));
#85365=CARTESIAN_POINT('Ctrl Pts',(448.590917961239,-26.0126948878623,26.0126948878623));
#85366=CARTESIAN_POINT('Ctrl Pts',(448.590917961239,-26.0126948878623,0.));
#85367=CARTESIAN_POINT('Ctrl Pts',(448.590917961239,-26.0126948878623,-26.0126948878623));
#85368=CARTESIAN_POINT('Ctrl Pts',(448.590917961239,0.,-26.0126948878623));
#85369=CARTESIAN_POINT('Ctrl Pts',(448.590917961239,26.0126948878623,-26.0126948878623));
#85370=CARTESIAN_POINT('Ctrl Pts',(448.590917961239,26.0126948878623,0.));
#85371=CARTESIAN_POINT('Ctrl Pts',(447.957393443862,24.9479052384017,0.));
#85372=CARTESIAN_POINT('Ctrl Pts',(447.957393443862,24.9479052384016,24.9479052384016));
#85373=CARTESIAN_POINT('Ctrl Pts',(447.957393443862,0.,24.9479052384017));
#85374=CARTESIAN_POINT('Ctrl Pts',(447.957393443862,-24.9479052384016,24.9479052384016));
#85375=CARTESIAN_POINT('Ctrl Pts',(447.957393443862,-24.9479052384017,0.));
#85376=CARTESIAN_POINT('Ctrl Pts',(447.957393443862,-24.9479052384016,-24.9479052384016));
#85377=CARTESIAN_POINT('Ctrl Pts',(447.957393443862,0.,-24.9479052384017));
#85378=CARTESIAN_POINT('Ctrl Pts',(447.957393443862,24.9479052384016,-24.9479052384016));
#85379=CARTESIAN_POINT('Ctrl Pts',(447.957393443862,24.9479052384017,0.));
#85380=CARTESIAN_POINT('Ctrl Pts',(447.33053455453,23.8059316147879,0.));
#85381=CARTESIAN_POINT('Ctrl Pts',(447.33053455453,23.8059316147879,23.8059316147879));
#85382=CARTESIAN_POINT('Ctrl Pts',(447.33053455453,0.,23.8059316147879));
#85383=CARTESIAN_POINT('Ctrl Pts',(447.33053455453,-23.8059316147879,23.8059316147879));
#85384=CARTESIAN_POINT('Ctrl Pts',(447.33053455453,-23.8059316147879,0.));
#85385=CARTESIAN_POINT('Ctrl Pts',(447.33053455453,-23.8059316147879,-23.8059316147879));
#85386=CARTESIAN_POINT('Ctrl Pts',(447.33053455453,0.,-23.8059316147879));
#85387=CARTESIAN_POINT('Ctrl Pts',(447.33053455453,23.8059316147879,-23.8059316147879));
#85388=CARTESIAN_POINT('Ctrl Pts',(447.33053455453,23.8059316147879,0.));
#85389=CARTESIAN_POINT('Ctrl Pts',(446.701568257837,22.648007840472,0.));
#85390=CARTESIAN_POINT('Ctrl Pts',(446.701568257837,22.648007840472,22.648007840472));
#85391=CARTESIAN_POINT('Ctrl Pts',(446.701568257837,0.,22.648007840472));
#85392=CARTESIAN_POINT('Ctrl Pts',(446.701568257837,-22.648007840472,22.648007840472));
#85393=CARTESIAN_POINT('Ctrl Pts',(446.701568257837,-22.648007840472,0.));
#85394=CARTESIAN_POINT('Ctrl Pts',(446.701568257837,-22.648007840472,-22.648007840472));
#85395=CARTESIAN_POINT('Ctrl Pts',(446.701568257837,0.,-22.648007840472));
#85396=CARTESIAN_POINT('Ctrl Pts',(446.701568257837,22.648007840472,-22.648007840472));
#85397=CARTESIAN_POINT('Ctrl Pts',(446.701568257837,22.648007840472,0.));
#85398=CARTESIAN_POINT('Ctrl Pts',(446.063094810897,21.5522443018912,0.));
#85399=CARTESIAN_POINT('Ctrl Pts',(446.063094810897,21.5522443018912,21.5522443018912));
#85400=CARTESIAN_POINT('Ctrl Pts',(446.063094810897,0.,21.5522443018912));
#85401=CARTESIAN_POINT('Ctrl Pts',(446.063094810897,-21.5522443018912,21.5522443018912));
#85402=CARTESIAN_POINT('Ctrl Pts',(446.063094810897,-21.5522443018912,0.));
#85403=CARTESIAN_POINT('Ctrl Pts',(446.063094810897,-21.5522443018912,-21.5522443018912));
#85404=CARTESIAN_POINT('Ctrl Pts',(446.063094810897,0.,-21.5522443018912));
#85405=CARTESIAN_POINT('Ctrl Pts',(446.063094810897,21.5522443018912,-21.5522443018912));
#85406=CARTESIAN_POINT('Ctrl Pts',(446.063094810897,21.5522443018912,0.));
#85407=CARTESIAN_POINT('Ctrl Pts',(445.409724117899,20.6026006224608,0.));
#85408=CARTESIAN_POINT('Ctrl Pts',(445.409724117899,20.6026006224608,20.6026006224608));
#85409=CARTESIAN_POINT('Ctrl Pts',(445.409724117899,0.,20.6026006224608));
#85410=CARTESIAN_POINT('Ctrl Pts',(445.409724117899,-20.6026006224608,20.6026006224608));
#85411=CARTESIAN_POINT('Ctrl Pts',(445.409724117899,-20.6026006224608,0.));
#85412=CARTESIAN_POINT('Ctrl Pts',(445.409724117899,-20.6026006224608,-20.6026006224608));
#85413=CARTESIAN_POINT('Ctrl Pts',(445.409724117899,0.,-20.6026006224608));
#85414=CARTESIAN_POINT('Ctrl Pts',(445.409724117899,20.6026006224608,-20.6026006224608));
#85415=CARTESIAN_POINT('Ctrl Pts',(445.409724117899,20.6026006224608,0.));
#85416=CARTESIAN_POINT('Ctrl Pts',(444.738673713096,19.8775193263257,0.));
#85417=CARTESIAN_POINT('Ctrl Pts',(444.738673713096,19.8775193263257,19.8775193263257));
#85418=CARTESIAN_POINT('Ctrl Pts',(444.738673713096,0.,19.8775193263257));
#85419=CARTESIAN_POINT('Ctrl Pts',(444.738673713096,-19.8775193263257,19.8775193263257));
#85420=CARTESIAN_POINT('Ctrl Pts',(444.738673713096,-19.8775193263257,0.));
#85421=CARTESIAN_POINT('Ctrl Pts',(444.738673713096,-19.8775193263257,-19.8775193263257));
#85422=CARTESIAN_POINT('Ctrl Pts',(444.738673713096,0.,-19.8775193263257));
#85423=CARTESIAN_POINT('Ctrl Pts',(444.738673713096,19.8775193263257,-19.8775193263257));
#85424=CARTESIAN_POINT('Ctrl Pts',(444.738673713096,19.8775193263257,0.));
#85425=CARTESIAN_POINT('Ctrl Pts',(444.050403766182,19.4385599502075,0.));
#85426=CARTESIAN_POINT('Ctrl Pts',(444.050403766182,19.4385599502075,19.4385599502075));
#85427=CARTESIAN_POINT('Ctrl Pts',(444.050403766182,0.,19.4385599502075));
#85428=CARTESIAN_POINT('Ctrl Pts',(444.050403766182,-19.4385599502075,19.4385599502075));
#85429=CARTESIAN_POINT('Ctrl Pts',(444.050403766182,-19.4385599502075,0.));
#85430=CARTESIAN_POINT('Ctrl Pts',(444.050403766182,-19.4385599502075,-19.4385599502075));
#85431=CARTESIAN_POINT('Ctrl Pts',(444.050403766182,0.,-19.4385599502075));
#85432=CARTESIAN_POINT('Ctrl Pts',(444.050403766182,19.4385599502075,-19.4385599502075));
#85433=CARTESIAN_POINT('Ctrl Pts',(444.050403766182,19.4385599502075,0.));
#85434=CARTESIAN_POINT('Ctrl Pts',(443.349192839921,19.3193585552553,0.));
#85435=CARTESIAN_POINT('Ctrl Pts',(443.349192839921,19.3193585552553,19.3193585552553));
#85436=CARTESIAN_POINT('Ctrl Pts',(443.349192839921,0.,19.3193585552553));
#85437=CARTESIAN_POINT('Ctrl Pts',(443.349192839921,-19.3193585552553,19.3193585552553));
#85438=CARTESIAN_POINT('Ctrl Pts',(443.349192839921,-19.3193585552553,0.));
#85439=CARTESIAN_POINT('Ctrl Pts',(443.349192839921,-19.3193585552553,-19.3193585552553));
#85440=CARTESIAN_POINT('Ctrl Pts',(443.349192839921,0.,-19.3193585552553));
#85441=CARTESIAN_POINT('Ctrl Pts',(443.349192839921,19.3193585552553,-19.3193585552553));
#85442=CARTESIAN_POINT('Ctrl Pts',(443.349192839921,19.3193585552553,0.));
#85443=CARTESIAN_POINT('Ctrl Pts',(442.643867874371,19.5135261763159,0.));
#85444=CARTESIAN_POINT('Ctrl Pts',(442.643867874371,19.5135261763159,19.5135261763159));
#85445=CARTESIAN_POINT('Ctrl Pts',(442.643867874371,0.,19.5135261763159));
#85446=CARTESIAN_POINT('Ctrl Pts',(442.643867874371,-19.5135261763159,19.5135261763159));
#85447=CARTESIAN_POINT('Ctrl Pts',(442.643867874371,-19.5135261763159,0.));
#85448=CARTESIAN_POINT('Ctrl Pts',(442.643867874371,-19.5135261763159,-19.5135261763159));
#85449=CARTESIAN_POINT('Ctrl Pts',(442.643867874371,0.,-19.5135261763159));
#85450=CARTESIAN_POINT('Ctrl Pts',(442.643867874371,19.5135261763159,-19.5135261763159));
#85451=CARTESIAN_POINT('Ctrl Pts',(442.643867874371,19.5135261763159,0.));
#85452=CARTESIAN_POINT('Ctrl Pts',(441.945455216616,19.9815541289552,0.));
#85453=CARTESIAN_POINT('Ctrl Pts',(441.945455216616,19.9815541289552,19.9815541289552));
#85454=CARTESIAN_POINT('Ctrl Pts',(441.945455216616,0.,19.9815541289552));
#85455=CARTESIAN_POINT('Ctrl Pts',(441.945455216616,-19.9815541289552,19.9815541289552));
#85456=CARTESIAN_POINT('Ctrl Pts',(441.945455216616,-19.9815541289552,0.));
#85457=CARTESIAN_POINT('Ctrl Pts',(441.945455216616,-19.9815541289552,-19.9815541289552));
#85458=CARTESIAN_POINT('Ctrl Pts',(441.945455216616,0.,-19.9815541289552));
#85459=CARTESIAN_POINT('Ctrl Pts',(441.945455216616,19.9815541289552,-19.9815541289552));
#85460=CARTESIAN_POINT('Ctrl Pts',(441.945455216616,19.9815541289552,0.));
#85461=CARTESIAN_POINT('Ctrl Pts',(441.264476356928,20.6589404895745,0.));
#85462=CARTESIAN_POINT('Ctrl Pts',(441.264476356928,20.6589404895745,20.6589404895745));
#85463=CARTESIAN_POINT('Ctrl Pts',(441.264476356928,0.,20.6589404895745));
#85464=CARTESIAN_POINT('Ctrl Pts',(441.264476356928,-20.6589404895745,20.6589404895745));
#85465=CARTESIAN_POINT('Ctrl Pts',(441.264476356928,-20.6589404895745,0.));
#85466=CARTESIAN_POINT('Ctrl Pts',(441.264476356928,-20.6589404895745,-20.6589404895745));
#85467=CARTESIAN_POINT('Ctrl Pts',(441.264476356928,0.,-20.6589404895745));
#85468=CARTESIAN_POINT('Ctrl Pts',(441.264476356928,20.6589404895745,-20.6589404895745));
#85469=CARTESIAN_POINT('Ctrl Pts',(441.264476356928,20.6589404895745,0.));
#85470=CARTESIAN_POINT('Ctrl Pts',(440.608663208255,21.4639316820362,0.));
#85471=CARTESIAN_POINT('Ctrl Pts',(440.608663208255,21.4639316820362,21.4639316820362));
#85472=CARTESIAN_POINT('Ctrl Pts',(440.608663208255,0.,21.4639316820362));
#85473=CARTESIAN_POINT('Ctrl Pts',(440.608663208255,-21.4639316820362,21.4639316820362));
#85474=CARTESIAN_POINT('Ctrl Pts',(440.608663208255,-21.4639316820362,0.));
#85475=CARTESIAN_POINT('Ctrl Pts',(440.608663208255,-21.4639316820362,-21.4639316820362));
#85476=CARTESIAN_POINT('Ctrl Pts',(440.608663208255,0.,-21.4639316820362));
#85477=CARTESIAN_POINT('Ctrl Pts',(440.608663208255,21.4639316820362,-21.4639316820362));
#85478=CARTESIAN_POINT('Ctrl Pts',(440.608663208255,21.4639316820362,0.));
#85479=CARTESIAN_POINT('Ctrl Pts',(439.979788998029,22.3052361760555,0.));
#85480=CARTESIAN_POINT('Ctrl Pts',(439.979788998029,22.3052361760555,22.3052361760555));
#85481=CARTESIAN_POINT('Ctrl Pts',(439.979788998029,0.,22.3052361760555));
#85482=CARTESIAN_POINT('Ctrl Pts',(439.979788998029,-22.3052361760555,22.3052361760555));
#85483=CARTESIAN_POINT('Ctrl Pts',(439.979788998029,-22.3052361760555,0.));
#85484=CARTESIAN_POINT('Ctrl Pts',(439.979788998029,-22.3052361760555,-22.3052361760555));
#85485=CARTESIAN_POINT('Ctrl Pts',(439.979788998029,0.,-22.3052361760555));
#85486=CARTESIAN_POINT('Ctrl Pts',(439.979788998029,22.3052361760555,-22.3052361760555));
#85487=CARTESIAN_POINT('Ctrl Pts',(439.979788998029,22.3052361760555,0.));
#85488=CARTESIAN_POINT('Ctrl Pts',(439.374041195168,23.0904544768451,0.));
#85489=CARTESIAN_POINT('Ctrl Pts',(439.374041195168,23.0904544768451,23.0904544768451));
#85490=CARTESIAN_POINT('Ctrl Pts',(439.374041195168,0.,23.0904544768451));
#85491=CARTESIAN_POINT('Ctrl Pts',(439.374041195168,-23.0904544768451,23.0904544768451));
#85492=CARTESIAN_POINT('Ctrl Pts',(439.374041195168,-23.0904544768451,0.));
#85493=CARTESIAN_POINT('Ctrl Pts',(439.374041195168,-23.0904544768451,-23.0904544768451));
#85494=CARTESIAN_POINT('Ctrl Pts',(439.374041195168,0.,-23.0904544768451));
#85495=CARTESIAN_POINT('Ctrl Pts',(439.374041195168,23.0904544768451,-23.0904544768451));
#85496=CARTESIAN_POINT('Ctrl Pts',(439.374041195168,23.0904544768451,0.));
#85497=CARTESIAN_POINT('Ctrl Pts',(438.784711462182,23.7347409739043,0.));
#85498=CARTESIAN_POINT('Ctrl Pts',(438.784711462182,23.7347409739043,23.7347409739043));
#85499=CARTESIAN_POINT('Ctrl Pts',(438.784711462182,0.,23.7347409739043));
#85500=CARTESIAN_POINT('Ctrl Pts',(438.784711462182,-23.7347409739043,23.7347409739043));
#85501=CARTESIAN_POINT('Ctrl Pts',(438.784711462182,-23.7347409739043,0.));
#85502=CARTESIAN_POINT('Ctrl Pts',(438.784711462182,-23.7347409739043,-23.7347409739043));
#85503=CARTESIAN_POINT('Ctrl Pts',(438.784711462182,0.,-23.7347409739043));
#85504=CARTESIAN_POINT('Ctrl Pts',(438.784711462182,23.7347409739043,-23.7347409739043));
#85505=CARTESIAN_POINT('Ctrl Pts',(438.784711462182,23.7347409739043,0.));
#85506=CARTESIAN_POINT('Ctrl Pts',(438.204301429719,24.169942753537,0.));
#85507=CARTESIAN_POINT('Ctrl Pts',(438.204301429719,24.169942753537,24.169942753537));
#85508=CARTESIAN_POINT('Ctrl Pts',(438.204301429719,0.,24.169942753537));
#85509=CARTESIAN_POINT('Ctrl Pts',(438.204301429719,-24.169942753537,24.169942753537));
#85510=CARTESIAN_POINT('Ctrl Pts',(438.204301429719,-24.169942753537,0.));
#85511=CARTESIAN_POINT('Ctrl Pts',(438.204301429719,-24.169942753537,-24.169942753537));
#85512=CARTESIAN_POINT('Ctrl Pts',(438.204301429719,0.,-24.169942753537));
#85513=CARTESIAN_POINT('Ctrl Pts',(438.204301429719,24.169942753537,-24.169942753537));
#85514=CARTESIAN_POINT('Ctrl Pts',(438.204301429719,24.169942753537,0.));
#85515=CARTESIAN_POINT('Ctrl Pts',(437.626635727528,24.3523414078208,0.));
#85516=CARTESIAN_POINT('Ctrl Pts',(437.626635727528,24.3523414078208,24.3523414078208));
#85517=CARTESIAN_POINT('Ctrl Pts',(437.626635727528,0.,24.3523414078208));
#85518=CARTESIAN_POINT('Ctrl Pts',(437.626635727528,-24.3523414078208,24.3523414078208));
#85519=CARTESIAN_POINT('Ctrl Pts',(437.626635727528,-24.3523414078208,0.));
#85520=CARTESIAN_POINT('Ctrl Pts',(437.626635727528,-24.3523414078208,-24.3523414078208));
#85521=CARTESIAN_POINT('Ctrl Pts',(437.626635727528,0.,-24.3523414078208));
#85522=CARTESIAN_POINT('Ctrl Pts',(437.626635727528,24.3523414078208,-24.3523414078208));
#85523=CARTESIAN_POINT('Ctrl Pts',(437.626635727528,24.3523414078208,0.));
#85524=CARTESIAN_POINT('Ctrl Pts',(437.049555721009,24.2740379737108,0.));
#85525=CARTESIAN_POINT('Ctrl Pts',(437.049555721009,24.2740379737108,24.2740379737108));
#85526=CARTESIAN_POINT('Ctrl Pts',(437.049555721009,0.,24.2740379737108));
#85527=CARTESIAN_POINT('Ctrl Pts',(437.049555721009,-24.2740379737108,24.2740379737108));
#85528=CARTESIAN_POINT('Ctrl Pts',(437.049555721009,-24.2740379737108,0.));
#85529=CARTESIAN_POINT('Ctrl Pts',(437.049555721009,-24.2740379737108,-24.2740379737108));
#85530=CARTESIAN_POINT('Ctrl Pts',(437.049555721009,0.,-24.2740379737108));
#85531=CARTESIAN_POINT('Ctrl Pts',(437.049555721009,24.2740379737108,-24.2740379737108));
#85532=CARTESIAN_POINT('Ctrl Pts',(437.049555721009,24.2740379737108,0.));
#85533=CARTESIAN_POINT('Ctrl Pts',(436.47446919765,23.9577550832877,0.));
#85534=CARTESIAN_POINT('Ctrl Pts',(436.47446919765,23.9577550832877,23.9577550832877));
#85535=CARTESIAN_POINT('Ctrl Pts',(436.47446919765,0.,23.9577550832877));
#85536=CARTESIAN_POINT('Ctrl Pts',(436.47446919765,-23.9577550832877,23.9577550832877));
#85537=CARTESIAN_POINT('Ctrl Pts',(436.47446919765,-23.9577550832877,0.));
#85538=CARTESIAN_POINT('Ctrl Pts',(436.47446919765,-23.9577550832877,-23.9577550832877));
#85539=CARTESIAN_POINT('Ctrl Pts',(436.47446919765,0.,-23.9577550832877));
#85540=CARTESIAN_POINT('Ctrl Pts',(436.47446919765,23.9577550832877,-23.9577550832877));
#85541=CARTESIAN_POINT('Ctrl Pts',(436.47446919765,23.9577550832877,0.));
#85542=CARTESIAN_POINT('Ctrl Pts',(435.90424315295,23.4431754196512,0.));
#85543=CARTESIAN_POINT('Ctrl Pts',(435.90424315295,23.4431754196512,23.4431754196512));
#85544=CARTESIAN_POINT('Ctrl Pts',(435.90424315295,0.,23.4431754196512));
#85545=CARTESIAN_POINT('Ctrl Pts',(435.90424315295,-23.4431754196512,23.4431754196512));
#85546=CARTESIAN_POINT('Ctrl Pts',(435.90424315295,-23.4431754196512,0.));
#85547=CARTESIAN_POINT('Ctrl Pts',(435.90424315295,-23.4431754196512,-23.4431754196512));
#85548=CARTESIAN_POINT('Ctrl Pts',(435.90424315295,0.,-23.4431754196512));
#85549=CARTESIAN_POINT('Ctrl Pts',(435.90424315295,23.4431754196512,-23.4431754196512));
#85550=CARTESIAN_POINT('Ctrl Pts',(435.90424315295,23.4431754196512,0.));
#85551=CARTESIAN_POINT('Ctrl Pts',(435.341499781773,22.7752920967055,0.));
#85552=CARTESIAN_POINT('Ctrl Pts',(435.341499781773,22.7752920967055,22.7752920967055));
#85553=CARTESIAN_POINT('Ctrl Pts',(435.341499781773,0.,22.7752920967055));
#85554=CARTESIAN_POINT('Ctrl Pts',(435.341499781773,-22.7752920967055,22.7752920967055));
#85555=CARTESIAN_POINT('Ctrl Pts',(435.341499781773,-22.7752920967055,0.));
#85556=CARTESIAN_POINT('Ctrl Pts',(435.341499781773,-22.7752920967055,-22.7752920967055));
#85557=CARTESIAN_POINT('Ctrl Pts',(435.341499781773,0.,-22.7752920967055));
#85558=CARTESIAN_POINT('Ctrl Pts',(435.341499781773,22.7752920967055,-22.7752920967055));
#85559=CARTESIAN_POINT('Ctrl Pts',(435.341499781773,22.7752920967055,0.));
#85560=CARTESIAN_POINT('Ctrl Pts',(434.787071478856,21.9937093229656,0.));
#85561=CARTESIAN_POINT('Ctrl Pts',(434.787071478856,21.9937093229656,21.9937093229656));
#85562=CARTESIAN_POINT('Ctrl Pts',(434.787071478856,0.,21.9937093229656));
#85563=CARTESIAN_POINT('Ctrl Pts',(434.787071478856,-21.9937093229656,21.9937093229656));
#85564=CARTESIAN_POINT('Ctrl Pts',(434.787071478856,-21.9937093229656,0.));
#85565=CARTESIAN_POINT('Ctrl Pts',(434.787071478856,-21.9937093229656,-21.9937093229656));
#85566=CARTESIAN_POINT('Ctrl Pts',(434.787071478856,0.,-21.9937093229656));
#85567=CARTESIAN_POINT('Ctrl Pts',(434.787071478856,21.9937093229656,-21.9937093229656));
#85568=CARTESIAN_POINT('Ctrl Pts',(434.787071478856,21.9937093229656,0.));
#85569=CARTESIAN_POINT('Ctrl Pts',(434.240615161377,21.1336209998616,0.));
#85570=CARTESIAN_POINT('Ctrl Pts',(434.240615161377,21.1336209998616,21.1336209998616));
#85571=CARTESIAN_POINT('Ctrl Pts',(434.240615161377,0.,21.1336209998616));
#85572=CARTESIAN_POINT('Ctrl Pts',(434.240615161377,-21.1336209998616,21.1336209998616));
#85573=CARTESIAN_POINT('Ctrl Pts',(434.240615161377,-21.1336209998616,0.));
#85574=CARTESIAN_POINT('Ctrl Pts',(434.240615161377,-21.1336209998616,-21.1336209998616));
#85575=CARTESIAN_POINT('Ctrl Pts',(434.240615161377,0.,-21.1336209998616));
#85576=CARTESIAN_POINT('Ctrl Pts',(434.240615161377,21.1336209998616,-21.1336209998616));
#85577=CARTESIAN_POINT('Ctrl Pts',(434.240615161377,21.1336209998616,0.));
#85578=CARTESIAN_POINT('Ctrl Pts',(433.700924533454,20.2252100813003,0.));
#85579=CARTESIAN_POINT('Ctrl Pts',(433.700924533454,20.2252100813003,20.2252100813003));
#85580=CARTESIAN_POINT('Ctrl Pts',(433.700924533454,0.,20.2252100813003));
#85581=CARTESIAN_POINT('Ctrl Pts',(433.700924533454,-20.2252100813003,20.2252100813003));
#85582=CARTESIAN_POINT('Ctrl Pts',(433.700924533454,-20.2252100813003,0.));
#85583=CARTESIAN_POINT('Ctrl Pts',(433.700924533454,-20.2252100813003,-20.2252100813003));
#85584=CARTESIAN_POINT('Ctrl Pts',(433.700924533454,0.,-20.2252100813003));
#85585=CARTESIAN_POINT('Ctrl Pts',(433.700924533454,20.2252100813003,-20.2252100813003));
#85586=CARTESIAN_POINT('Ctrl Pts',(433.700924533454,20.2252100813003,0.));
#85587=CARTESIAN_POINT('Ctrl Pts',(433.16637200178,19.2936381483974,0.));
#85588=CARTESIAN_POINT('Ctrl Pts',(433.16637200178,19.2936381483973,19.2936381483973));
#85589=CARTESIAN_POINT('Ctrl Pts',(433.16637200178,0.,19.2936381483974));
#85590=CARTESIAN_POINT('Ctrl Pts',(433.16637200178,-19.2936381483973,19.2936381483973));
#85591=CARTESIAN_POINT('Ctrl Pts',(433.16637200178,-19.2936381483974,0.));
#85592=CARTESIAN_POINT('Ctrl Pts',(433.16637200178,-19.2936381483973,-19.2936381483973));
#85593=CARTESIAN_POINT('Ctrl Pts',(433.16637200178,0.,-19.2936381483974));
#85594=CARTESIAN_POINT('Ctrl Pts',(433.16637200178,19.2936381483973,-19.2936381483973));
#85595=CARTESIAN_POINT('Ctrl Pts',(433.16637200178,19.2936381483974,0.));
#85596=CARTESIAN_POINT('Ctrl Pts',(432.635268474333,18.3588432671141,0.));
#85597=CARTESIAN_POINT('Ctrl Pts',(432.635268474333,18.3588432671141,18.3588432671141));
#85598=CARTESIAN_POINT('Ctrl Pts',(432.635268474333,0.,18.3588432671141));
#85599=CARTESIAN_POINT('Ctrl Pts',(432.635268474333,-18.3588432671141,18.3588432671141));
#85600=CARTESIAN_POINT('Ctrl Pts',(432.635268474333,-18.3588432671141,0.));
#85601=CARTESIAN_POINT('Ctrl Pts',(432.635268474333,-18.3588432671141,-18.3588432671141));
#85602=CARTESIAN_POINT('Ctrl Pts',(432.635268474333,0.,-18.3588432671141));
#85603=CARTESIAN_POINT('Ctrl Pts',(432.635268474333,18.3588432671141,-18.3588432671141));
#85604=CARTESIAN_POINT('Ctrl Pts',(432.635268474333,18.3588432671141,0.));
#85605=CARTESIAN_POINT('Ctrl Pts',(432.10632569174,17.4352566594404,0.));
#85606=CARTESIAN_POINT('Ctrl Pts',(432.10632569174,17.4352566594404,17.4352566594404));
#85607=CARTESIAN_POINT('Ctrl Pts',(432.10632569174,0.,17.4352566594404));
#85608=CARTESIAN_POINT('Ctrl Pts',(432.10632569174,-17.4352566594404,17.4352566594404));
#85609=CARTESIAN_POINT('Ctrl Pts',(432.10632569174,-17.4352566594404,0.));
#85610=CARTESIAN_POINT('Ctrl Pts',(432.10632569174,-17.4352566594404,-17.4352566594404));
#85611=CARTESIAN_POINT('Ctrl Pts',(432.10632569174,0.,-17.4352566594404));
#85612=CARTESIAN_POINT('Ctrl Pts',(432.10632569174,17.4352566594404,-17.4352566594404));
#85613=CARTESIAN_POINT('Ctrl Pts',(432.10632569174,17.4352566594404,0.));
#85614=CARTESIAN_POINT('Ctrl Pts',(431.578706159811,16.5324288334304,0.));
#85615=CARTESIAN_POINT('Ctrl Pts',(431.578706159811,16.5324288334304,16.5324288334304));
#85616=CARTESIAN_POINT('Ctrl Pts',(431.578706159811,0.,16.5324288334304));
#85617=CARTESIAN_POINT('Ctrl Pts',(431.578706159811,-16.5324288334304,16.5324288334304));
#85618=CARTESIAN_POINT('Ctrl Pts',(431.578706159811,-16.5324288334304,0.));
#85619=CARTESIAN_POINT('Ctrl Pts',(431.578706159811,-16.5324288334304,-16.5324288334304));
#85620=CARTESIAN_POINT('Ctrl Pts',(431.578706159811,0.,-16.5324288334304));
#85621=CARTESIAN_POINT('Ctrl Pts',(431.578706159811,16.5324288334304,-16.5324288334304));
#85622=CARTESIAN_POINT('Ctrl Pts',(431.578706159811,16.5324288334304,0.));
#85623=CARTESIAN_POINT('Ctrl Pts',(431.051899252967,15.6560989394055,0.));
#85624=CARTESIAN_POINT('Ctrl Pts',(431.051899252967,15.6560989394055,15.6560989394055));
#85625=CARTESIAN_POINT('Ctrl Pts',(431.051899252967,0.,15.6560989394055));
#85626=CARTESIAN_POINT('Ctrl Pts',(431.051899252967,-15.6560989394055,15.6560989394055));
#85627=CARTESIAN_POINT('Ctrl Pts',(431.051899252967,-15.6560989394055,0.));
#85628=CARTESIAN_POINT('Ctrl Pts',(431.051899252967,-15.6560989394055,-15.6560989394055));
#85629=CARTESIAN_POINT('Ctrl Pts',(431.051899252967,0.,-15.6560989394055));
#85630=CARTESIAN_POINT('Ctrl Pts',(431.051899252967,15.6560989394055,-15.6560989394055));
#85631=CARTESIAN_POINT('Ctrl Pts',(431.051899252967,15.6560989394055,0.));
#85632=CARTESIAN_POINT('Ctrl Pts',(430.630902033383,14.9785137687881,0.));
#85633=CARTESIAN_POINT('Ctrl Pts',(430.630902033383,14.9785137687881,14.9785137687881));
#85634=CARTESIAN_POINT('Ctrl Pts',(430.630902033383,0.,14.9785137687881));
#85635=CARTESIAN_POINT('Ctrl Pts',(430.630902033383,-14.9785137687881,14.9785137687881));
#85636=CARTESIAN_POINT('Ctrl Pts',(430.630902033383,-14.9785137687881,0.));
#85637=CARTESIAN_POINT('Ctrl Pts',(430.630902033383,-14.9785137687881,-14.9785137687881));
#85638=CARTESIAN_POINT('Ctrl Pts',(430.630902033383,0.,-14.9785137687881));
#85639=CARTESIAN_POINT('Ctrl Pts',(430.630902033383,14.9785137687881,-14.9785137687881));
#85640=CARTESIAN_POINT('Ctrl Pts',(430.630902033383,14.9785137687881,0.));
#85641=CARTESIAN_POINT('Ctrl Pts',(430.315367854661,14.4839565936731,0.));
#85642=CARTESIAN_POINT('Ctrl Pts',(430.315367854661,14.4839565936731,14.4839565936731));
#85643=CARTESIAN_POINT('Ctrl Pts',(430.315367854661,0.,14.4839565936731));
#85644=CARTESIAN_POINT('Ctrl Pts',(430.315367854661,-14.4839565936731,14.4839565936731));
#85645=CARTESIAN_POINT('Ctrl Pts',(430.315367854661,-14.4839565936731,0.));
#85646=CARTESIAN_POINT('Ctrl Pts',(430.315367854661,-14.4839565936731,-14.4839565936731));
#85647=CARTESIAN_POINT('Ctrl Pts',(430.315367854661,0.,-14.4839565936731));
#85648=CARTESIAN_POINT('Ctrl Pts',(430.315367854661,14.4839565936731,-14.4839565936731));
#85649=CARTESIAN_POINT('Ctrl Pts',(430.315367854661,14.4839565936731,0.));
#85650=CARTESIAN_POINT('Ctrl Pts',(430.105106779965,14.1603092797614,0.));
#85651=CARTESIAN_POINT('Ctrl Pts',(430.105106779965,14.1603092797614,14.1603092797614));
#85652=CARTESIAN_POINT('Ctrl Pts',(430.105106779965,0.,14.1603092797614));
#85653=CARTESIAN_POINT('Ctrl Pts',(430.105106779965,-14.1603092797614,14.1603092797614));
#85654=CARTESIAN_POINT('Ctrl Pts',(430.105106779965,-14.1603092797614,0.));
#85655=CARTESIAN_POINT('Ctrl Pts',(430.105106779965,-14.1603092797614,-14.1603092797614));
#85656=CARTESIAN_POINT('Ctrl Pts',(430.105106779965,0.,-14.1603092797614));
#85657=CARTESIAN_POINT('Ctrl Pts',(430.105106779965,14.1603092797614,-14.1603092797614));
#85658=CARTESIAN_POINT('Ctrl Pts',(430.105106779965,14.1603092797614,0.));
#85659=CARTESIAN_POINT('Ctrl Pts',(430.,14.,0.));
#85660=CARTESIAN_POINT('Ctrl Pts',(430.,14.,14.));
#85661=CARTESIAN_POINT('Ctrl Pts',(430.,0.,14.));
#85662=CARTESIAN_POINT('Ctrl Pts',(430.,-14.,14.));
#85663=CARTESIAN_POINT('Ctrl Pts',(430.,-14.,0.));
#85664=CARTESIAN_POINT('Ctrl Pts',(430.,-14.,-14.));
#85665=CARTESIAN_POINT('Ctrl Pts',(430.,0.,-14.));
#85666=CARTESIAN_POINT('Ctrl Pts',(430.,14.,-14.));
#85667=CARTESIAN_POINT('Ctrl Pts',(430.,14.,0.));
#85668=CARTESIAN_POINT('',(498.,43.,0.));
#85669=CARTESIAN_POINT('Ctrl Pts',(430.,14.,0.));
#85670=CARTESIAN_POINT('Ctrl Pts',(430.105106779965,14.1603092797614,0.));
#85671=CARTESIAN_POINT('Ctrl Pts',(430.315367854661,14.4839565936731,0.));
#85672=CARTESIAN_POINT('Ctrl Pts',(430.630902033383,14.9785137687881,0.));
#85673=CARTESIAN_POINT('Ctrl Pts',(431.051899252967,15.6560989394055,0.));
#85674=CARTESIAN_POINT('Ctrl Pts',(431.578706159811,16.5324288334304,0.));
#85675=CARTESIAN_POINT('Ctrl Pts',(432.10632569174,17.4352566594404,0.));
#85676=CARTESIAN_POINT('Ctrl Pts',(432.635268474333,18.3588432671141,0.));
#85677=CARTESIAN_POINT('Ctrl Pts',(433.16637200178,19.2936381483974,0.));
#85678=CARTESIAN_POINT('Ctrl Pts',(433.700924533454,20.2252100813003,0.));
#85679=CARTESIAN_POINT('Ctrl Pts',(434.240615161377,21.1336209998616,0.));
#85680=CARTESIAN_POINT('Ctrl Pts',(434.787071478856,21.9937093229656,0.));
#85681=CARTESIAN_POINT('Ctrl Pts',(435.341499781773,22.7752920967055,0.));
#85682=CARTESIAN_POINT('Ctrl Pts',(435.90424315295,23.4431754196512,0.));
#85683=CARTESIAN_POINT('Ctrl Pts',(436.47446919765,23.9577550832877,0.));
#85684=CARTESIAN_POINT('Ctrl Pts',(437.049555721009,24.2740379737108,0.));
#85685=CARTESIAN_POINT('Ctrl Pts',(437.626635727528,24.3523414078208,0.));
#85686=CARTESIAN_POINT('Ctrl Pts',(438.204301429719,24.169942753537,0.));
#85687=CARTESIAN_POINT('Ctrl Pts',(438.784711462182,23.7347409739043,0.));
#85688=CARTESIAN_POINT('Ctrl Pts',(439.374041195168,23.0904544768451,0.));
#85689=CARTESIAN_POINT('Ctrl Pts',(439.979788998029,22.3052361760555,0.));
#85690=CARTESIAN_POINT('Ctrl Pts',(440.608663208255,21.4639316820362,0.));
#85691=CARTESIAN_POINT('Ctrl Pts',(441.264476356928,20.6589404895745,0.));
#85692=CARTESIAN_POINT('Ctrl Pts',(441.945455216616,19.9815541289552,0.));
#85693=CARTESIAN_POINT('Ctrl Pts',(442.643867874371,19.5135261763159,0.));
#85694=CARTESIAN_POINT('Ctrl Pts',(443.349192839921,19.3193585552553,0.));
#85695=CARTESIAN_POINT('Ctrl Pts',(444.050403766182,19.4385599502075,0.));
#85696=CARTESIAN_POINT('Ctrl Pts',(444.738673713096,19.8775193263257,0.));
#85697=CARTESIAN_POINT('Ctrl Pts',(445.409724117899,20.6026006224608,0.));
#85698=CARTESIAN_POINT('Ctrl Pts',(446.063094810897,21.5522443018912,0.));
#85699=CARTESIAN_POINT('Ctrl Pts',(446.701568257837,22.648007840472,0.));
#85700=CARTESIAN_POINT('Ctrl Pts',(447.33053455453,23.8059316147879,0.));
#85701=CARTESIAN_POINT('Ctrl Pts',(447.957393443862,24.9479052384017,0.));
#85702=CARTESIAN_POINT('Ctrl Pts',(448.590917961239,26.0126948878623,0.));
#85703=CARTESIAN_POINT('Ctrl Pts',(449.240699204464,26.9680450110966,0.));
#85704=CARTESIAN_POINT('Ctrl Pts',(449.91530974049,27.8028078305578,0.));
#85705=CARTESIAN_POINT('Ctrl Pts',(450.6204304333,28.5179209746754,0.));
#85706=CARTESIAN_POINT('Ctrl Pts',(451.356904731652,29.117599269821,0.));
#85707=CARTESIAN_POINT('Ctrl Pts',(452.119011172215,29.6009203712207,0.));
#85708=CARTESIAN_POINT('Ctrl Pts',(452.892185119924,29.9520957467627,0.));
#85709=CARTESIAN_POINT('Ctrl Pts',(453.65232362069,30.1347085607613,0.));
#85710=CARTESIAN_POINT('Ctrl Pts',(454.374221692176,30.1089010904408,0.));
#85711=CARTESIAN_POINT('Ctrl Pts',(455.038839374707,29.8456839543521,0.));
#85712=CARTESIAN_POINT('Ctrl Pts',(455.641185904649,29.3426365369257,0.));
#85713=CARTESIAN_POINT('Ctrl Pts',(456.197496723491,28.6382733820605,0.));
#85714=CARTESIAN_POINT('Ctrl Pts',(456.736386522373,27.8005738327045,0.));
#85715=CARTESIAN_POINT('Ctrl Pts',(457.290615845749,26.9163263890247,0.));
#85716=CARTESIAN_POINT('Ctrl Pts',(457.888379201951,26.0800747021197,0.));
#85717=CARTESIAN_POINT('Ctrl Pts',(458.545378831534,25.3834939706622,0.));
#85718=CARTESIAN_POINT('Ctrl Pts',(459.255007342274,24.9039206717732,0.));
#85719=CARTESIAN_POINT('Ctrl Pts',(459.994949810424,24.6992460116247,0.));
#85720=CARTESIAN_POINT('Ctrl Pts',(460.736933199464,24.8033903723626,0.));
#85721=CARTESIAN_POINT('Ctrl Pts',(461.454649264338,25.2224382685937,0.));
#85722=CARTESIAN_POINT('Ctrl Pts',(462.134199633467,25.9283453171447,0.));
#85723=CARTESIAN_POINT('Ctrl Pts',(462.775015619175,26.8639618331474,0.));
#85724=CARTESIAN_POINT('Ctrl Pts',(463.38544807492,27.9547399267918,0.));
#85725=CARTESIAN_POINT('Ctrl Pts',(463.980012926408,29.1182237614132,0.));
#85726=CARTESIAN_POINT('Ctrl Pts',(464.575897029354,30.2747905161882,0.));
#85727=CARTESIAN_POINT('Ctrl Pts',(465.189920345436,31.3570687154993,0.));
#85728=CARTESIAN_POINT('Ctrl Pts',(465.834971562565,32.3218329216103,0.));
#85729=CARTESIAN_POINT('Ctrl Pts',(466.517752610425,33.1545694480525,0.));
#85730=CARTESIAN_POINT('Ctrl Pts',(467.239271643519,33.8574930279435,0.));
#85731=CARTESIAN_POINT('Ctrl Pts',(467.994839856681,34.4411672254374,0.));
#85732=CARTESIAN_POINT('Ctrl Pts',(468.774141019888,34.9141595380048,0.));
#85733=CARTESIAN_POINT('Ctrl Pts',(469.561546477286,35.2747783728489,0.));
#85734=CARTESIAN_POINT('Ctrl Pts',(470.335597351742,35.4987206841576,0.));
#85735=CARTESIAN_POINT('Ctrl Pts',(471.073330047455,35.547602310438,0.));
#85736=CARTESIAN_POINT('Ctrl Pts',(471.756985572081,35.3862684299237,0.));
#85737=CARTESIAN_POINT('Ctrl Pts',(472.379062231055,34.9957749951357,0.));
#85738=CARTESIAN_POINT('Ctrl Pts',(472.950173506317,34.3917148430238,0.));
#85739=CARTESIAN_POINT('Ctrl Pts',(473.496207150892,33.6242325832595,0.));
#85740=CARTESIAN_POINT('Ctrl Pts',(474.048807350844,32.7664588883108,0.));
#85741=CARTESIAN_POINT('Ctrl Pts',(474.637420315231,31.9063742772383,0.));
#85742=CARTESIAN_POINT('Ctrl Pts',(475.281638153934,31.1373046376156,0.));
#85743=CARTESIAN_POINT('Ctrl Pts',(475.981110865709,30.5489260877444,0.));
#85744=CARTESIAN_POINT('Ctrl Pts',(476.715088006725,30.2182781872629,0.));
#85745=CARTESIAN_POINT('Ctrl Pts',(477.454558588677,30.2006533599419,0.));
#85746=CARTESIAN_POINT('Ctrl Pts',(478.170705434033,30.5212549544916,0.));
#85747=CARTESIAN_POINT('Ctrl Pts',(478.845896061198,31.1648170165913,0.));
#85748=CARTESIAN_POINT('Ctrl Pts',(479.480404754155,32.0713081103475,0.));
#85749=CARTESIAN_POINT('Ctrl Pts',(480.086198305556,33.1532218206079,0.));
#85750=CARTESIAN_POINT('Ctrl Pts',(480.682720968628,34.3094577320604,0.));
#85751=CARTESIAN_POINT('Ctrl Pts',(481.291935021843,35.4403955291427,0.));
#85752=CARTESIAN_POINT('Ctrl Pts',(481.933610981183,36.4627634902989,0.));
#85753=CARTESIAN_POINT('Ctrl Pts',(482.620675064127,37.3238846021003,0.));
#85754=CARTESIAN_POINT('Ctrl Pts',(483.354083971076,38.0181299396445,0.));
#85755=CARTESIAN_POINT('Ctrl Pts',(484.125459941715,38.5707804214382,0.));
#85756=CARTESIAN_POINT('Ctrl Pts',(484.9203435101,39.0198093895239,0.));
#85757=CARTESIAN_POINT('Ctrl Pts',(485.721282963476,39.3972368241277,0.));
#85758=CARTESIAN_POINT('Ctrl Pts',(486.510844647409,39.7133643175418,0.));
#85759=CARTESIAN_POINT('Ctrl Pts',(487.275021660065,39.9329323721432,0.));
#85760=CARTESIAN_POINT('Ctrl Pts',(488.00470898085,39.9896159368436,0.));
#85761=CARTESIAN_POINT('Ctrl Pts',(488.696302016509,39.8235950753685,0.));
#85762=CARTESIAN_POINT('Ctrl Pts',(489.35228088106,39.4079242082379,0.));
#85763=CARTESIAN_POINT('Ctrl Pts',(489.982486856253,38.7890664196497,0.));
#85764=CARTESIAN_POINT('Ctrl Pts',(490.602330907815,38.0826279556129,0.));
#85765=CARTESIAN_POINT('Ctrl Pts',(491.228327780497,37.4320007627789,0.));
#85766=CARTESIAN_POINT('Ctrl Pts',(491.874247942463,36.9763167796813,0.));
#85767=CARTESIAN_POINT('Ctrl Pts',(492.547316355638,36.8168662015777,0.));
#85768=CARTESIAN_POINT('Ctrl Pts',(493.243601186251,36.978223468014,0.));
#85769=CARTESIAN_POINT('Ctrl Pts',(493.950613427123,37.4232171946361,0.));
#85770=CARTESIAN_POINT('Ctrl Pts',(494.651570478316,38.080336648354,0.));
#85771=CARTESIAN_POINT('Ctrl Pts',(495.328808380576,38.8651538927084,0.));
#85772=CARTESIAN_POINT('Ctrl Pts',(495.968194348492,39.7081288650878,0.));
#85773=CARTESIAN_POINT('Ctrl Pts',(496.560639185004,40.5647779062035,0.));
#85774=CARTESIAN_POINT('Ctrl Pts',(497.100596959865,41.4077471164017,0.));
#85775=CARTESIAN_POINT('Ctrl Pts',(497.488406157359,42.0604608545242,0.));
#85776=CARTESIAN_POINT('Ctrl Pts',(497.754018276443,42.5357609366511,0.));
#85777=CARTESIAN_POINT('Ctrl Pts',(497.919875683486,42.8463072547191,0.));
#85778=CARTESIAN_POINT('Ctrl Pts',(498.,43.,0.));
#85779=CARTESIAN_POINT('',(498.,-43.,-5.26598123633362E-15));
#85780=CARTESIAN_POINT('Origin',(498.,0.,0.));
#85781=CARTESIAN_POINT('Origin',(498.,0.,0.));
#85782=CARTESIAN_POINT('Origin',(507.,0.,0.));
#85783=CARTESIAN_POINT('',(516.,-43.,-5.26598123633362E-15));
#85784=CARTESIAN_POINT('Origin',(516.,0.,0.));
#85785=CARTESIAN_POINT('',(507.,-43.,-5.26598123633362E-15));
#85786=CARTESIAN_POINT('Origin',(516.,41.,0.));
#85787=CARTESIAN_POINT('',(516.,-41.,-5.02105187650415E-15));
#85788=CARTESIAN_POINT('Origin',(516.,0.,0.));
#85789=CARTESIAN_POINT('Origin',(507.3,0.,0.));
#85790=CARTESIAN_POINT('',(498.6,-41.,-5.02105187650415E-15));
#85791=CARTESIAN_POINT('',(507.3,-41.,-5.02105187650415E-15));
#85792=CARTESIAN_POINT('Origin',(498.6,0.,0.));
#85793=CARTESIAN_POINT('Origin',(498.,0.,0.));
#85794=CARTESIAN_POINT('',(497.4,-40.,-4.89858719658941E-15));
#85795=CARTESIAN_POINT('',(498.,-40.5,-4.95981953654678E-15));
#85796=CARTESIAN_POINT('',(497.4,40.,0.));
#85797=CARTESIAN_POINT('Origin',(497.4,0.,0.));
#85798=CARTESIAN_POINT('Origin',(497.4,0.,0.));
#85799=CARTESIAN_POINT('Ctrl Pts',(431.,13.5,0.));
#85800=CARTESIAN_POINT('Ctrl Pts',(431.,13.5,13.5));
#85801=CARTESIAN_POINT('Ctrl Pts',(431.,0.,13.5));
#85802=CARTESIAN_POINT('Ctrl Pts',(431.,-13.5,13.5));
#85803=CARTESIAN_POINT('Ctrl Pts',(431.,-13.5,0.));
#85804=CARTESIAN_POINT('Ctrl Pts',(431.,-13.5,-13.5));
#85805=CARTESIAN_POINT('Ctrl Pts',(431.,0.,-13.5));
#85806=CARTESIAN_POINT('Ctrl Pts',(431.,13.5,-13.5));
#85807=CARTESIAN_POINT('Ctrl Pts',(431.,13.5,0.));
#85808=CARTESIAN_POINT('Ctrl Pts',(431.075930488729,13.5913677105967,0.));
#85809=CARTESIAN_POINT('Ctrl Pts',(431.075930488729,13.5913677105967,13.5913677105967));
#85810=CARTESIAN_POINT('Ctrl Pts',(431.075930488729,0.,13.5913677105967));
#85811=CARTESIAN_POINT('Ctrl Pts',(431.075930488729,-13.5913677105967,13.5913677105967));
#85812=CARTESIAN_POINT('Ctrl Pts',(431.075930488729,-13.5913677105967,0.));
#85813=CARTESIAN_POINT('Ctrl Pts',(431.075930488729,-13.5913677105967,-13.5913677105967));
#85814=CARTESIAN_POINT('Ctrl Pts',(431.075930488729,0.,-13.5913677105967));
#85815=CARTESIAN_POINT('Ctrl Pts',(431.075930488729,13.5913677105967,-13.5913677105967));
#85816=CARTESIAN_POINT('Ctrl Pts',(431.075930488729,13.5913677105967,0.));
#85817=CARTESIAN_POINT('Ctrl Pts',(431.230394288423,13.7832480588419,0.));
#85818=CARTESIAN_POINT('Ctrl Pts',(431.230394288423,13.7832480588419,13.7832480588419));
#85819=CARTESIAN_POINT('Ctrl Pts',(431.230394288423,0.,13.7832480588419));
#85820=CARTESIAN_POINT('Ctrl Pts',(431.230394288423,-13.7832480588419,13.7832480588419));
#85821=CARTESIAN_POINT('Ctrl Pts',(431.230394288423,-13.7832480588419,0.));
#85822=CARTESIAN_POINT('Ctrl Pts',(431.230394288423,-13.7832480588419,-13.7832480588419));
#85823=CARTESIAN_POINT('Ctrl Pts',(431.230394288423,0.,-13.7832480588419));
#85824=CARTESIAN_POINT('Ctrl Pts',(431.230394288423,13.7832480588419,-13.7832480588419));
#85825=CARTESIAN_POINT('Ctrl Pts',(431.230394288423,13.7832480588419,0.));
#85826=CARTESIAN_POINT('Ctrl Pts',(431.469898541327,14.0985040583044,0.));
#85827=CARTESIAN_POINT('Ctrl Pts',(431.469898541327,14.0985040583044,14.0985040583044));
#85828=CARTESIAN_POINT('Ctrl Pts',(431.469898541327,0.,14.0985040583044));
#85829=CARTESIAN_POINT('Ctrl Pts',(431.469898541327,-14.0985040583044,14.0985040583044));
#85830=CARTESIAN_POINT('Ctrl Pts',(431.469898541327,-14.0985040583044,0.));
#85831=CARTESIAN_POINT('Ctrl Pts',(431.469898541327,-14.0985040583044,-14.0985040583044));
#85832=CARTESIAN_POINT('Ctrl Pts',(431.469898541327,0.,-14.0985040583044));
#85833=CARTESIAN_POINT('Ctrl Pts',(431.469898541327,14.0985040583044,-14.0985040583044));
#85834=CARTESIAN_POINT('Ctrl Pts',(431.469898541327,14.0985040583044,0.));
#85835=CARTESIAN_POINT('Ctrl Pts',(431.804856206642,14.5737184153466,0.));
#85836=CARTESIAN_POINT('Ctrl Pts',(431.804856206642,14.5737184153466,14.5737184153466));
#85837=CARTESIAN_POINT('Ctrl Pts',(431.804856206642,0.,14.5737184153466));
#85838=CARTESIAN_POINT('Ctrl Pts',(431.804856206642,-14.5737184153466,14.5737184153466));
#85839=CARTESIAN_POINT('Ctrl Pts',(431.804856206642,-14.5737184153466,0.));
#85840=CARTESIAN_POINT('Ctrl Pts',(431.804856206642,-14.5737184153466,-14.5737184153466));
#85841=CARTESIAN_POINT('Ctrl Pts',(431.804856206642,0.,-14.5737184153466));
#85842=CARTESIAN_POINT('Ctrl Pts',(431.804856206642,14.5737184153466,-14.5737184153466));
#85843=CARTESIAN_POINT('Ctrl Pts',(431.804856206642,14.5737184153466,0.));
#85844=CARTESIAN_POINT('Ctrl Pts',(432.249367015116,15.2569713036193,0.));
#85845=CARTESIAN_POINT('Ctrl Pts',(432.249367015116,15.2569713036193,15.2569713036193));
#85846=CARTESIAN_POINT('Ctrl Pts',(432.249367015116,0.,15.2569713036193));
#85847=CARTESIAN_POINT('Ctrl Pts',(432.249367015116,-15.2569713036193,15.2569713036193));
#85848=CARTESIAN_POINT('Ctrl Pts',(432.249367015116,-15.2569713036193,0.));
#85849=CARTESIAN_POINT('Ctrl Pts',(432.249367015116,-15.2569713036193,-15.2569713036193));
#85850=CARTESIAN_POINT('Ctrl Pts',(432.249367015116,0.,-15.2569713036193));
#85851=CARTESIAN_POINT('Ctrl Pts',(432.249367015116,15.2569713036193,-15.2569713036193));
#85852=CARTESIAN_POINT('Ctrl Pts',(432.249367015116,15.2569713036193,0.));
#85853=CARTESIAN_POINT('Ctrl Pts',(432.719002234035,16.0226042712625,0.));
#85854=CARTESIAN_POINT('Ctrl Pts',(432.719002234035,16.0226042712625,16.0226042712625));
#85855=CARTESIAN_POINT('Ctrl Pts',(432.719002234035,0.,16.0226042712625));
#85856=CARTESIAN_POINT('Ctrl Pts',(432.719002234035,-16.0226042712625,16.0226042712625));
#85857=CARTESIAN_POINT('Ctrl Pts',(432.719002234035,-16.0226042712625,0.));
#85858=CARTESIAN_POINT('Ctrl Pts',(432.719002234035,-16.0226042712625,-16.0226042712625));
#85859=CARTESIAN_POINT('Ctrl Pts',(432.719002234035,0.,-16.0226042712625));
#85860=CARTESIAN_POINT('Ctrl Pts',(432.719002234035,16.0226042712625,-16.0226042712625));
#85861=CARTESIAN_POINT('Ctrl Pts',(432.719002234035,16.0226042712625,0.));
#85862=CARTESIAN_POINT('Ctrl Pts',(433.212390321051,16.8570423033932,0.));
#85863=CARTESIAN_POINT('Ctrl Pts',(433.212390321051,16.8570423033931,16.8570423033931));
#85864=CARTESIAN_POINT('Ctrl Pts',(433.212390321051,0.,16.8570423033932));
#85865=CARTESIAN_POINT('Ctrl Pts',(433.212390321051,-16.8570423033931,16.8570423033931));
#85866=CARTESIAN_POINT('Ctrl Pts',(433.212390321051,-16.8570423033932,0.));
#85867=CARTESIAN_POINT('Ctrl Pts',(433.212390321051,-16.8570423033931,-16.8570423033931));
#85868=CARTESIAN_POINT('Ctrl Pts',(433.212390321051,0.,-16.8570423033932));
#85869=CARTESIAN_POINT('Ctrl Pts',(433.212390321051,16.8570423033931,-16.8570423033931));
#85870=CARTESIAN_POINT('Ctrl Pts',(433.212390321051,16.8570423033932,0.));
#85871=CARTESIAN_POINT('Ctrl Pts',(433.727172908933,17.7371471664815,0.));
#85872=CARTESIAN_POINT('Ctrl Pts',(433.727172908933,17.7371471664815,17.7371471664815));
#85873=CARTESIAN_POINT('Ctrl Pts',(433.727172908933,0.,17.7371471664815));
#85874=CARTESIAN_POINT('Ctrl Pts',(433.727172908933,-17.7371471664815,17.7371471664815));
#85875=CARTESIAN_POINT('Ctrl Pts',(433.727172908933,-17.7371471664815,0.));
#85876=CARTESIAN_POINT('Ctrl Pts',(433.727172908933,-17.7371471664815,-17.7371471664815));
#85877=CARTESIAN_POINT('Ctrl Pts',(433.727172908933,0.,-17.7371471664815));
#85878=CARTESIAN_POINT('Ctrl Pts',(433.727172908933,17.7371471664815,-17.7371471664815));
#85879=CARTESIAN_POINT('Ctrl Pts',(433.727172908933,17.7371471664815,0.));
#85880=CARTESIAN_POINT('Ctrl Pts',(434.260020980134,18.6299473105583,0.));
#85881=CARTESIAN_POINT('Ctrl Pts',(434.260020980134,18.6299473105583,18.6299473105583));
#85882=CARTESIAN_POINT('Ctrl Pts',(434.260020980134,0.,18.6299473105583));
#85883=CARTESIAN_POINT('Ctrl Pts',(434.260020980134,-18.6299473105583,18.6299473105583));
#85884=CARTESIAN_POINT('Ctrl Pts',(434.260020980134,-18.6299473105583,0.));
#85885=CARTESIAN_POINT('Ctrl Pts',(434.260020980134,-18.6299473105583,-18.6299473105583));
#85886=CARTESIAN_POINT('Ctrl Pts',(434.260020980134,0.,-18.6299473105583));
#85887=CARTESIAN_POINT('Ctrl Pts',(434.260020980134,18.6299473105583,-18.6299473105583));
#85888=CARTESIAN_POINT('Ctrl Pts',(434.260020980134,18.6299473105583,0.));
#85889=CARTESIAN_POINT('Ctrl Pts',(434.807068105737,19.4956986413733,0.));
#85890=CARTESIAN_POINT('Ctrl Pts',(434.807068105737,19.4956986413733,19.4956986413733));
#85891=CARTESIAN_POINT('Ctrl Pts',(434.807068105737,0.,19.4956986413733));
#85892=CARTESIAN_POINT('Ctrl Pts',(434.807068105737,-19.4956986413733,19.4956986413733));
#85893=CARTESIAN_POINT('Ctrl Pts',(434.807068105737,-19.4956986413733,0.));
#85894=CARTESIAN_POINT('Ctrl Pts',(434.807068105737,-19.4956986413733,-19.4956986413733));
#85895=CARTESIAN_POINT('Ctrl Pts',(434.807068105737,0.,-19.4956986413733));
#85896=CARTESIAN_POINT('Ctrl Pts',(434.807068105737,19.4956986413733,-19.4956986413733));
#85897=CARTESIAN_POINT('Ctrl Pts',(434.807068105737,19.4956986413733,0.));
#85898=CARTESIAN_POINT('Ctrl Pts',(435.364242124671,20.2901523149136,0.));
#85899=CARTESIAN_POINT('Ctrl Pts',(435.364242124671,20.2901523149136,20.2901523149136));
#85900=CARTESIAN_POINT('Ctrl Pts',(435.364242124671,0.,20.2901523149136));
#85901=CARTESIAN_POINT('Ctrl Pts',(435.364242124671,-20.2901523149136,20.2901523149136));
#85902=CARTESIAN_POINT('Ctrl Pts',(435.364242124671,-20.2901523149136,0.));
#85903=CARTESIAN_POINT('Ctrl Pts',(435.364242124671,-20.2901523149136,-20.2901523149136));
#85904=CARTESIAN_POINT('Ctrl Pts',(435.364242124671,0.,-20.2901523149136));
#85905=CARTESIAN_POINT('Ctrl Pts',(435.364242124671,20.2901523149136,-20.2901523149136));
#85906=CARTESIAN_POINT('Ctrl Pts',(435.364242124671,20.2901523149136,0.));
#85907=CARTESIAN_POINT('Ctrl Pts',(435.927631335713,20.9670478075204,0.));
#85908=CARTESIAN_POINT('Ctrl Pts',(435.927631335713,20.9670478075204,20.9670478075204));
#85909=CARTESIAN_POINT('Ctrl Pts',(435.927631335713,0.,20.9670478075204));
#85910=CARTESIAN_POINT('Ctrl Pts',(435.927631335713,-20.9670478075204,20.9670478075204));
#85911=CARTESIAN_POINT('Ctrl Pts',(435.927631335713,-20.9670478075204,0.));
#85912=CARTESIAN_POINT('Ctrl Pts',(435.927631335713,-20.9670478075204,-20.9670478075204));
#85913=CARTESIAN_POINT('Ctrl Pts',(435.927631335713,0.,-20.9670478075204));
#85914=CARTESIAN_POINT('Ctrl Pts',(435.927631335713,20.9670478075204,-20.9670478075204));
#85915=CARTESIAN_POINT('Ctrl Pts',(435.927631335713,20.9670478075204,0.));
#85916=CARTESIAN_POINT('Ctrl Pts',(436.493850849539,21.4807238935623,0.));
#85917=CARTESIAN_POINT('Ctrl Pts',(436.493850849539,21.4807238935623,21.4807238935623));
#85918=CARTESIAN_POINT('Ctrl Pts',(436.493850849539,0.,21.4807238935623));
#85919=CARTESIAN_POINT('Ctrl Pts',(436.493850849539,-21.4807238935623,21.4807238935623));
#85920=CARTESIAN_POINT('Ctrl Pts',(436.493850849539,-21.4807238935623,0.));
#85921=CARTESIAN_POINT('Ctrl Pts',(436.493850849539,-21.4807238935623,-21.4807238935623));
#85922=CARTESIAN_POINT('Ctrl Pts',(436.493850849539,0.,-21.4807238935623));
#85923=CARTESIAN_POINT('Ctrl Pts',(436.493850849539,21.4807238935623,-21.4807238935623));
#85924=CARTESIAN_POINT('Ctrl Pts',(436.493850849539,21.4807238935623,0.));
#85925=CARTESIAN_POINT('Ctrl Pts',(437.060372222462,21.7881221006031,0.));
#85926=CARTESIAN_POINT('Ctrl Pts',(437.060372222462,21.7881221006031,21.7881221006031));
#85927=CARTESIAN_POINT('Ctrl Pts',(437.060372222462,0.,21.7881221006031));
#85928=CARTESIAN_POINT('Ctrl Pts',(437.060372222462,-21.7881221006031,21.7881221006031));
#85929=CARTESIAN_POINT('Ctrl Pts',(437.060372222462,-21.7881221006031,0.));
#85930=CARTESIAN_POINT('Ctrl Pts',(437.060372222462,-21.7881221006031,-21.7881221006031));
#85931=CARTESIAN_POINT('Ctrl Pts',(437.060372222462,0.,-21.7881221006031));
#85932=CARTESIAN_POINT('Ctrl Pts',(437.060372222462,21.7881221006031,-21.7881221006031));
#85933=CARTESIAN_POINT('Ctrl Pts',(437.060372222462,21.7881221006031,0.));
#85934=CARTESIAN_POINT('Ctrl Pts',(437.62612331768,21.8564147928601,0.));
#85935=CARTESIAN_POINT('Ctrl Pts',(437.62612331768,21.8564147928601,21.8564147928601));
#85936=CARTESIAN_POINT('Ctrl Pts',(437.62612331768,0.,21.8564147928601));
#85937=CARTESIAN_POINT('Ctrl Pts',(437.62612331768,-21.8564147928601,21.8564147928601));
#85938=CARTESIAN_POINT('Ctrl Pts',(437.62612331768,-21.8564147928601,0.));
#85939=CARTESIAN_POINT('Ctrl Pts',(437.62612331768,-21.8564147928601,-21.8564147928601));
#85940=CARTESIAN_POINT('Ctrl Pts',(437.62612331768,0.,-21.8564147928601));
#85941=CARTESIAN_POINT('Ctrl Pts',(437.62612331768,21.8564147928601,-21.8564147928601));
#85942=CARTESIAN_POINT('Ctrl Pts',(437.62612331768,21.8564147928601,0.));
#85943=CARTESIAN_POINT('Ctrl Pts',(438.191994671,21.6705685715134,0.));
#85944=CARTESIAN_POINT('Ctrl Pts',(438.191994671,21.6705685715134,21.6705685715134));
#85945=CARTESIAN_POINT('Ctrl Pts',(438.191994671,0.,21.6705685715134));
#85946=CARTESIAN_POINT('Ctrl Pts',(438.191994671,-21.6705685715134,21.6705685715134));
#85947=CARTESIAN_POINT('Ctrl Pts',(438.191994671,-21.6705685715134,0.));
#85948=CARTESIAN_POINT('Ctrl Pts',(438.191994671,-21.6705685715134,-21.6705685715134));
#85949=CARTESIAN_POINT('Ctrl Pts',(438.191994671,0.,-21.6705685715134));
#85950=CARTESIAN_POINT('Ctrl Pts',(438.191994671,21.6705685715134,-21.6705685715134));
#85951=CARTESIAN_POINT('Ctrl Pts',(438.191994671,21.6705685715134,0.));
#85952=CARTESIAN_POINT('Ctrl Pts',(438.761636765821,21.2425737573923,0.));
#85953=CARTESIAN_POINT('Ctrl Pts',(438.761636765821,21.2425737573923,21.2425737573923));
#85954=CARTESIAN_POINT('Ctrl Pts',(438.761636765821,0.,21.2425737573923));
#85955=CARTESIAN_POINT('Ctrl Pts',(438.761636765821,-21.2425737573923,21.2425737573923));
#85956=CARTESIAN_POINT('Ctrl Pts',(438.761636765821,-21.2425737573923,0.));
#85957=CARTESIAN_POINT('Ctrl Pts',(438.761636765821,-21.2425737573923,-21.2425737573923));
#85958=CARTESIAN_POINT('Ctrl Pts',(438.761636765821,0.,-21.2425737573923));
#85959=CARTESIAN_POINT('Ctrl Pts',(438.761636765821,21.2425737573923,-21.2425737573923));
#85960=CARTESIAN_POINT('Ctrl Pts',(438.761636765821,21.2425737573923,0.));
#85961=CARTESIAN_POINT('Ctrl Pts',(439.341309422512,20.6146885506738,0.));
#85962=CARTESIAN_POINT('Ctrl Pts',(439.341309422512,20.6146885506738,20.6146885506738));
#85963=CARTESIAN_POINT('Ctrl Pts',(439.341309422512,0.,20.6146885506738));
#85964=CARTESIAN_POINT('Ctrl Pts',(439.341309422512,-20.6146885506738,20.6146885506738));
#85965=CARTESIAN_POINT('Ctrl Pts',(439.341309422512,-20.6146885506738,0.));
#85966=CARTESIAN_POINT('Ctrl Pts',(439.341309422512,-20.6146885506738,-20.6146885506738));
#85967=CARTESIAN_POINT('Ctrl Pts',(439.341309422512,0.,-20.6146885506738));
#85968=CARTESIAN_POINT('Ctrl Pts',(439.341309422512,20.6146885506738,-20.6146885506738));
#85969=CARTESIAN_POINT('Ctrl Pts',(439.341309422512,20.6146885506738,0.));
#85970=CARTESIAN_POINT('Ctrl Pts',(439.937886180109,19.8503961731823,0.));
#85971=CARTESIAN_POINT('Ctrl Pts',(439.937886180109,19.8503961731823,19.8503961731823));
#85972=CARTESIAN_POINT('Ctrl Pts',(439.937886180109,0.,19.8503961731823));
#85973=CARTESIAN_POINT('Ctrl Pts',(439.937886180109,-19.8503961731823,19.8503961731823));
#85974=CARTESIAN_POINT('Ctrl Pts',(439.937886180109,-19.8503961731823,0.));
#85975=CARTESIAN_POINT('Ctrl Pts',(439.937886180109,-19.8503961731823,-19.8503961731823));
#85976=CARTESIAN_POINT('Ctrl Pts',(439.937886180109,0.,-19.8503961731823));
#85977=CARTESIAN_POINT('Ctrl Pts',(439.937886180109,19.8503961731823,-19.8503961731823));
#85978=CARTESIAN_POINT('Ctrl Pts',(439.937886180109,19.8503961731823,0.));
#85979=CARTESIAN_POINT('Ctrl Pts',(440.557174885988,19.0280111167061,0.));
#85980=CARTESIAN_POINT('Ctrl Pts',(440.557174885988,19.0280111167061,19.0280111167061));
#85981=CARTESIAN_POINT('Ctrl Pts',(440.557174885988,0.,19.0280111167061));
#85982=CARTESIAN_POINT('Ctrl Pts',(440.557174885988,-19.0280111167061,19.0280111167061));
#85983=CARTESIAN_POINT('Ctrl Pts',(440.557174885988,-19.0280111167061,0.));
#85984=CARTESIAN_POINT('Ctrl Pts',(440.557174885988,-19.0280111167061,-19.0280111167061));
#85985=CARTESIAN_POINT('Ctrl Pts',(440.557174885988,0.,-19.0280111167061));
#85986=CARTESIAN_POINT('Ctrl Pts',(440.557174885988,19.0280111167061,-19.0280111167061));
#85987=CARTESIAN_POINT('Ctrl Pts',(440.557174885988,19.0280111167061,0.));
#85988=CARTESIAN_POINT('Ctrl Pts',(441.202275420219,18.2332083062446,0.));
#85989=CARTESIAN_POINT('Ctrl Pts',(441.202275420219,18.2332083062446,18.2332083062446));
#85990=CARTESIAN_POINT('Ctrl Pts',(441.202275420219,0.,18.2332083062446));
#85991=CARTESIAN_POINT('Ctrl Pts',(441.202275420219,-18.2332083062446,18.2332083062446));
#85992=CARTESIAN_POINT('Ctrl Pts',(441.202275420219,-18.2332083062446,0.));
#85993=CARTESIAN_POINT('Ctrl Pts',(441.202275420219,-18.2332083062446,-18.2332083062446));
#85994=CARTESIAN_POINT('Ctrl Pts',(441.202275420219,0.,-18.2332083062446));
#85995=CARTESIAN_POINT('Ctrl Pts',(441.202275420219,18.2332083062446,-18.2332083062446));
#85996=CARTESIAN_POINT('Ctrl Pts',(441.202275420219,18.2332083062446,0.));
#85997=CARTESIAN_POINT('Ctrl Pts',(441.871528812589,17.5520839307903,0.));
#85998=CARTESIAN_POINT('Ctrl Pts',(441.871528812589,17.5520839307903,17.5520839307903));
#85999=CARTESIAN_POINT('Ctrl Pts',(441.871528812589,0.,17.5520839307903));
#86000=CARTESIAN_POINT('Ctrl Pts',(441.871528812589,-17.5520839307903,17.5520839307903));
#86001=CARTESIAN_POINT('Ctrl Pts',(441.871528812589,-17.5520839307903,0.));
#86002=CARTESIAN_POINT('Ctrl Pts',(441.871528812589,-17.5520839307903,-17.5520839307903));
#86003=CARTESIAN_POINT('Ctrl Pts',(441.871528812589,0.,-17.5520839307903));
#86004=CARTESIAN_POINT('Ctrl Pts',(441.871528812589,17.5520839307903,-17.5520839307903));
#86005=CARTESIAN_POINT('Ctrl Pts',(441.871528812589,17.5520839307903,0.));
#86006=CARTESIAN_POINT('Ctrl Pts',(442.557926874702,17.0637870913372,0.));
#86007=CARTESIAN_POINT('Ctrl Pts',(442.557926874702,17.0637870913372,17.0637870913372));
#86008=CARTESIAN_POINT('Ctrl Pts',(442.557926874702,0.,17.0637870913372));
#86009=CARTESIAN_POINT('Ctrl Pts',(442.557926874702,-17.0637870913372,17.0637870913372));
#86010=CARTESIAN_POINT('Ctrl Pts',(442.557926874702,-17.0637870913372,0.));
#86011=CARTESIAN_POINT('Ctrl Pts',(442.557926874702,-17.0637870913372,-17.0637870913372));
#86012=CARTESIAN_POINT('Ctrl Pts',(442.557926874702,0.,-17.0637870913372));
#86013=CARTESIAN_POINT('Ctrl Pts',(442.557926874702,17.0637870913372,-17.0637870913372));
#86014=CARTESIAN_POINT('Ctrl Pts',(442.557926874702,17.0637870913372,0.));
#86015=CARTESIAN_POINT('Ctrl Pts',(443.251810955599,16.8328795404879,0.));
#86016=CARTESIAN_POINT('Ctrl Pts',(443.251810955599,16.8328795404879,16.8328795404879));
#86017=CARTESIAN_POINT('Ctrl Pts',(443.251810955599,0.,16.8328795404879));
#86018=CARTESIAN_POINT('Ctrl Pts',(443.251810955599,-16.8328795404879,16.8328795404879));
#86019=CARTESIAN_POINT('Ctrl Pts',(443.251810955599,-16.8328795404879,0.));
#86020=CARTESIAN_POINT('Ctrl Pts',(443.251810955599,-16.8328795404879,-16.8328795404879));
#86021=CARTESIAN_POINT('Ctrl Pts',(443.251810955599,0.,-16.8328795404879));
#86022=CARTESIAN_POINT('Ctrl Pts',(443.251810955599,16.8328795404879,-16.8328795404879));
#86023=CARTESIAN_POINT('Ctrl Pts',(443.251810955599,16.8328795404879,0.));
#86024=CARTESIAN_POINT('Ctrl Pts',(443.942925321305,16.9015384494366,0.));
#86025=CARTESIAN_POINT('Ctrl Pts',(443.942925321305,16.9015384494366,16.9015384494366));
#86026=CARTESIAN_POINT('Ctrl Pts',(443.942925321305,0.,16.9015384494366));
#86027=CARTESIAN_POINT('Ctrl Pts',(443.942925321305,-16.9015384494366,16.9015384494366));
#86028=CARTESIAN_POINT('Ctrl Pts',(443.942925321305,-16.9015384494366,0.));
#86029=CARTESIAN_POINT('Ctrl Pts',(443.942925321305,-16.9015384494366,-16.9015384494366));
#86030=CARTESIAN_POINT('Ctrl Pts',(443.942925321305,0.,-16.9015384494366));
#86031=CARTESIAN_POINT('Ctrl Pts',(443.942925321305,16.9015384494366,-16.9015384494366));
#86032=CARTESIAN_POINT('Ctrl Pts',(443.942925321305,16.9015384494366,0.));
#86033=CARTESIAN_POINT('Ctrl Pts',(444.622665692905,17.2822090124047,0.));
#86034=CARTESIAN_POINT('Ctrl Pts',(444.622665692905,17.2822090124047,17.2822090124047));
#86035=CARTESIAN_POINT('Ctrl Pts',(444.622665692905,0.,17.2822090124047));
#86036=CARTESIAN_POINT('Ctrl Pts',(444.622665692905,-17.2822090124047,17.2822090124047));
#86037=CARTESIAN_POINT('Ctrl Pts',(444.622665692905,-17.2822090124047,0.));
#86038=CARTESIAN_POINT('Ctrl Pts',(444.622665692905,-17.2822090124047,-17.2822090124047));
#86039=CARTESIAN_POINT('Ctrl Pts',(444.622665692905,0.,-17.2822090124047));
#86040=CARTESIAN_POINT('Ctrl Pts',(444.622665692905,17.2822090124047,-17.2822090124047));
#86041=CARTESIAN_POINT('Ctrl Pts',(444.622665692905,17.2822090124047,0.));
#86042=CARTESIAN_POINT('Ctrl Pts',(445.286408098586,17.9489859823433,0.));
#86043=CARTESIAN_POINT('Ctrl Pts',(445.286408098586,17.9489859823433,17.9489859823433));
#86044=CARTESIAN_POINT('Ctrl Pts',(445.286408098586,0.,17.9489859823433));
#86045=CARTESIAN_POINT('Ctrl Pts',(445.286408098586,-17.9489859823433,17.9489859823433));
#86046=CARTESIAN_POINT('Ctrl Pts',(445.286408098586,-17.9489859823433,0.));
#86047=CARTESIAN_POINT('Ctrl Pts',(445.286408098586,-17.9489859823433,-17.9489859823433));
#86048=CARTESIAN_POINT('Ctrl Pts',(445.286408098586,0.,-17.9489859823433));
#86049=CARTESIAN_POINT('Ctrl Pts',(445.286408098586,17.9489859823433,-17.9489859823433));
#86050=CARTESIAN_POINT('Ctrl Pts',(445.286408098586,17.9489859823433,0.));
#86051=CARTESIAN_POINT('Ctrl Pts',(445.933164114128,18.8470019997588,0.));
#86052=CARTESIAN_POINT('Ctrl Pts',(445.933164114128,18.8470019997588,18.8470019997588));
#86053=CARTESIAN_POINT('Ctrl Pts',(445.933164114128,0.,18.8470019997588));
#86054=CARTESIAN_POINT('Ctrl Pts',(445.933164114128,-18.8470019997588,18.8470019997588));
#86055=CARTESIAN_POINT('Ctrl Pts',(445.933164114128,-18.8470019997588,0.));
#86056=CARTESIAN_POINT('Ctrl Pts',(445.933164114128,-18.8470019997588,-18.8470019997588));
#86057=CARTESIAN_POINT('Ctrl Pts',(445.933164114128,0.,-18.8470019997588));
#86058=CARTESIAN_POINT('Ctrl Pts',(445.933164114128,18.8470019997588,-18.8470019997588));
#86059=CARTESIAN_POINT('Ctrl Pts',(445.933164114128,18.8470019997588,0.));
#86060=CARTESIAN_POINT('Ctrl Pts',(446.564983118453,19.9034942867493,0.));
#86061=CARTESIAN_POINT('Ctrl Pts',(446.564983118453,19.9034942867493,19.9034942867493));
#86062=CARTESIAN_POINT('Ctrl Pts',(446.564983118453,0.,19.9034942867493));
#86063=CARTESIAN_POINT('Ctrl Pts',(446.564983118453,-19.9034942867493,19.9034942867493));
#86064=CARTESIAN_POINT('Ctrl Pts',(446.564983118453,-19.9034942867493,0.));
#86065=CARTESIAN_POINT('Ctrl Pts',(446.564983118453,-19.9034942867493,-19.9034942867493));
#86066=CARTESIAN_POINT('Ctrl Pts',(446.564983118453,0.,-19.9034942867493));
#86067=CARTESIAN_POINT('Ctrl Pts',(446.564983118453,19.9034942867493,-19.9034942867493));
#86068=CARTESIAN_POINT('Ctrl Pts',(446.564983118453,19.9034942867493,0.));
#86069=CARTESIAN_POINT('Ctrl Pts',(447.186436510144,21.0380603073665,0.));
#86070=CARTESIAN_POINT('Ctrl Pts',(447.186436510144,21.0380603073665,21.0380603073665));
#86071=CARTESIAN_POINT('Ctrl Pts',(447.186436510144,0.,21.0380603073665));
#86072=CARTESIAN_POINT('Ctrl Pts',(447.186436510144,-21.0380603073665,21.0380603073665));
#86073=CARTESIAN_POINT('Ctrl Pts',(447.186436510144,-21.0380603073665,0.));
#86074=CARTESIAN_POINT('Ctrl Pts',(447.186436510144,-21.0380603073665,-21.0380603073665));
#86075=CARTESIAN_POINT('Ctrl Pts',(447.186436510144,0.,-21.0380603073665));
#86076=CARTESIAN_POINT('Ctrl Pts',(447.186436510144,21.0380603073665,-21.0380603073665));
#86077=CARTESIAN_POINT('Ctrl Pts',(447.186436510144,21.0380603073665,0.));
#86078=CARTESIAN_POINT('Ctrl Pts',(447.804096970417,22.1736869588598,0.));
#86079=CARTESIAN_POINT('Ctrl Pts',(447.804096970417,22.1736869588598,22.1736869588598));
#86080=CARTESIAN_POINT('Ctrl Pts',(447.804096970417,0.,22.1736869588598));
#86081=CARTESIAN_POINT('Ctrl Pts',(447.804096970417,-22.1736869588598,22.1736869588598));
#86082=CARTESIAN_POINT('Ctrl Pts',(447.804096970417,-22.1736869588598,0.));
#86083=CARTESIAN_POINT('Ctrl Pts',(447.804096970417,-22.1736869588598,-22.1736869588598));
#86084=CARTESIAN_POINT('Ctrl Pts',(447.804096970417,0.,-22.1736869588598));
#86085=CARTESIAN_POINT('Ctrl Pts',(447.804096970417,22.1736869588598,-22.1736869588598));
#86086=CARTESIAN_POINT('Ctrl Pts',(447.804096970417,22.1736869588598,0.));
#86087=CARTESIAN_POINT('Ctrl Pts',(448.425955791819,23.2464235854324,0.));
#86088=CARTESIAN_POINT('Ctrl Pts',(448.425955791819,23.2464235854324,23.2464235854324));
#86089=CARTESIAN_POINT('Ctrl Pts',(448.425955791819,0.,23.2464235854324));
#86090=CARTESIAN_POINT('Ctrl Pts',(448.425955791819,-23.2464235854324,23.2464235854324));
#86091=CARTESIAN_POINT('Ctrl Pts',(448.425955791819,-23.2464235854324,0.));
#86092=CARTESIAN_POINT('Ctrl Pts',(448.425955791819,-23.2464235854324,-23.2464235854324));
#86093=CARTESIAN_POINT('Ctrl Pts',(448.425955791819,0.,-23.2464235854324));
#86094=CARTESIAN_POINT('Ctrl Pts',(448.425955791819,23.2464235854324,-23.2464235854324));
#86095=CARTESIAN_POINT('Ctrl Pts',(448.425955791819,23.2464235854324,0.));
#86096=CARTESIAN_POINT('Ctrl Pts',(449.061035117611,24.2182549404179,0.));
#86097=CARTESIAN_POINT('Ctrl Pts',(449.061035117611,24.2182549404179,24.2182549404179));
#86098=CARTESIAN_POINT('Ctrl Pts',(449.061035117611,0.,24.2182549404179));
#86099=CARTESIAN_POINT('Ctrl Pts',(449.061035117611,-24.2182549404179,24.2182549404179));
#86100=CARTESIAN_POINT('Ctrl Pts',(449.061035117611,-24.2182549404179,0.));
#86101=CARTESIAN_POINT('Ctrl Pts',(449.061035117611,-24.2182549404179,-24.2182549404179));
#86102=CARTESIAN_POINT('Ctrl Pts',(449.061035117611,0.,-24.2182549404179));
#86103=CARTESIAN_POINT('Ctrl Pts',(449.061035117611,24.2182549404179,-24.2182549404179));
#86104=CARTESIAN_POINT('Ctrl Pts',(449.061035117611,24.2182549404179,0.));
#86105=CARTESIAN_POINT('Ctrl Pts',(449.71798609425,25.074273116099,0.));
#86106=CARTESIAN_POINT('Ctrl Pts',(449.71798609425,25.074273116099,25.074273116099));
#86107=CARTESIAN_POINT('Ctrl Pts',(449.71798609425,0.,25.074273116099));
#86108=CARTESIAN_POINT('Ctrl Pts',(449.71798609425,-25.074273116099,25.074273116099));
#86109=CARTESIAN_POINT('Ctrl Pts',(449.71798609425,-25.074273116099,0.));
#86110=CARTESIAN_POINT('Ctrl Pts',(449.71798609425,-25.074273116099,-25.074273116099));
#86111=CARTESIAN_POINT('Ctrl Pts',(449.71798609425,0.,-25.074273116099));
#86112=CARTESIAN_POINT('Ctrl Pts',(449.71798609425,25.074273116099,-25.074273116099));
#86113=CARTESIAN_POINT('Ctrl Pts',(449.71798609425,25.074273116099,0.));
#86114=CARTESIAN_POINT('Ctrl Pts',(450.403201234375,25.8128681585372,0.));
#86115=CARTESIAN_POINT('Ctrl Pts',(450.403201234375,25.8128681585372,25.8128681585372));
#86116=CARTESIAN_POINT('Ctrl Pts',(450.403201234375,0.,25.8128681585372));
#86117=CARTESIAN_POINT('Ctrl Pts',(450.403201234375,-25.8128681585372,25.8128681585372));
#86118=CARTESIAN_POINT('Ctrl Pts',(450.403201234375,-25.8128681585372,0.));
#86119=CARTESIAN_POINT('Ctrl Pts',(450.403201234375,-25.8128681585372,-25.8128681585372));
#86120=CARTESIAN_POINT('Ctrl Pts',(450.403201234375,0.,-25.8128681585372));
#86121=CARTESIAN_POINT('Ctrl Pts',(450.403201234375,25.8128681585372,-25.8128681585372));
#86122=CARTESIAN_POINT('Ctrl Pts',(450.403201234375,25.8128681585372,0.));
#86123=CARTESIAN_POINT('Ctrl Pts',(451.119142458871,26.4383182927734,0.));
#86124=CARTESIAN_POINT('Ctrl Pts',(451.119142458871,26.4383182927734,26.4383182927734));
#86125=CARTESIAN_POINT('Ctrl Pts',(451.119142458871,0.,26.4383182927734));
#86126=CARTESIAN_POINT('Ctrl Pts',(451.119142458871,-26.4383182927734,26.4383182927734));
#86127=CARTESIAN_POINT('Ctrl Pts',(451.119142458871,-26.4383182927734,0.));
#86128=CARTESIAN_POINT('Ctrl Pts',(451.119142458871,-26.4383182927734,-26.4383182927734));
#86129=CARTESIAN_POINT('Ctrl Pts',(451.119142458871,0.,-26.4383182927734));
#86130=CARTESIAN_POINT('Ctrl Pts',(451.119142458871,26.4383182927734,-26.4383182927734));
#86131=CARTESIAN_POINT('Ctrl Pts',(451.119142458871,26.4383182927734,0.));
#86132=CARTESIAN_POINT('Ctrl Pts',(451.862441449957,26.9520337795735,0.));
#86133=CARTESIAN_POINT('Ctrl Pts',(451.862441449957,26.9520337795735,26.9520337795735));
#86134=CARTESIAN_POINT('Ctrl Pts',(451.862441449957,0.,26.9520337795735));
#86135=CARTESIAN_POINT('Ctrl Pts',(451.862441449957,-26.9520337795735,26.9520337795735));
#86136=CARTESIAN_POINT('Ctrl Pts',(451.862441449957,-26.9520337795735,0.));
#86137=CARTESIAN_POINT('Ctrl Pts',(451.862441449957,-26.9520337795735,-26.9520337795735));
#86138=CARTESIAN_POINT('Ctrl Pts',(451.862441449957,0.,-26.9520337795735));
#86139=CARTESIAN_POINT('Ctrl Pts',(451.862441449957,26.9520337795735,-26.9520337795735));
#86140=CARTESIAN_POINT('Ctrl Pts',(451.862441449957,26.9520337795735,0.));
#86141=CARTESIAN_POINT('Ctrl Pts',(452.622411993808,27.3452045659704,0.));
#86142=CARTESIAN_POINT('Ctrl Pts',(452.622411993808,27.3452045659704,27.3452045659704));
#86143=CARTESIAN_POINT('Ctrl Pts',(452.622411993808,0.,27.3452045659704));
#86144=CARTESIAN_POINT('Ctrl Pts',(452.622411993808,-27.3452045659704,27.3452045659704));
#86145=CARTESIAN_POINT('Ctrl Pts',(452.622411993808,-27.3452045659704,0.));
#86146=CARTESIAN_POINT('Ctrl Pts',(452.622411993808,-27.3452045659704,-27.3452045659704));
#86147=CARTESIAN_POINT('Ctrl Pts',(452.622411993808,0.,-27.3452045659704));
#86148=CARTESIAN_POINT('Ctrl Pts',(452.622411993808,27.3452045659704,-27.3452045659704));
#86149=CARTESIAN_POINT('Ctrl Pts',(452.622411993808,27.3452045659704,0.));
#86150=CARTESIAN_POINT('Ctrl Pts',(453.378537630885,27.5886555924961,0.));
#86151=CARTESIAN_POINT('Ctrl Pts',(453.378537630885,27.5886555924961,27.5886555924961));
#86152=CARTESIAN_POINT('Ctrl Pts',(453.378537630885,0.,27.5886555924961));
#86153=CARTESIAN_POINT('Ctrl Pts',(453.378537630885,-27.5886555924961,27.5886555924961));
#86154=CARTESIAN_POINT('Ctrl Pts',(453.378537630885,-27.5886555924961,0.));
#86155=CARTESIAN_POINT('Ctrl Pts',(453.378537630885,-27.5886555924961,-27.5886555924961));
#86156=CARTESIAN_POINT('Ctrl Pts',(453.378537630885,0.,-27.5886555924961));
#86157=CARTESIAN_POINT('Ctrl Pts',(453.378537630885,27.5886555924961,-27.5886555924961));
#86158=CARTESIAN_POINT('Ctrl Pts',(453.378537630885,27.5886555924961,0.));
#86159=CARTESIAN_POINT('Ctrl Pts',(454.106137134847,27.6435191850799,0.));
#86160=CARTESIAN_POINT('Ctrl Pts',(454.106137134847,27.6435191850799,27.6435191850799));
#86161=CARTESIAN_POINT('Ctrl Pts',(454.106137134847,0.,27.6435191850799));
#86162=CARTESIAN_POINT('Ctrl Pts',(454.106137134847,-27.6435191850799,27.6435191850799));
#86163=CARTESIAN_POINT('Ctrl Pts',(454.106137134847,-27.6435191850799,0.));
#86164=CARTESIAN_POINT('Ctrl Pts',(454.106137134847,-27.6435191850799,-27.6435191850799));
#86165=CARTESIAN_POINT('Ctrl Pts',(454.106137134847,0.,-27.6435191850799));
#86166=CARTESIAN_POINT('Ctrl Pts',(454.106137134847,27.6435191850799,-27.6435191850799));
#86167=CARTESIAN_POINT('Ctrl Pts',(454.106137134847,27.6435191850799,0.));
#86168=CARTESIAN_POINT('Ctrl Pts',(454.784171241843,27.4768576432717,0.));
#86169=CARTESIAN_POINT('Ctrl Pts',(454.784171241843,27.4768576432717,27.4768576432717));
#86170=CARTESIAN_POINT('Ctrl Pts',(454.784171241843,0.,27.4768576432717));
#86171=CARTESIAN_POINT('Ctrl Pts',(454.784171241843,-27.4768576432717,27.4768576432717));
#86172=CARTESIAN_POINT('Ctrl Pts',(454.784171241843,-27.4768576432717,0.));
#86173=CARTESIAN_POINT('Ctrl Pts',(454.784171241843,-27.4768576432717,-27.4768576432717));
#86174=CARTESIAN_POINT('Ctrl Pts',(454.784171241843,0.,-27.4768576432717));
#86175=CARTESIAN_POINT('Ctrl Pts',(454.784171241843,27.4768576432717,-27.4768576432717));
#86176=CARTESIAN_POINT('Ctrl Pts',(454.784171241843,27.4768576432717,0.));
#86177=CARTESIAN_POINT('Ctrl Pts',(455.401407401473,27.0741275496278,0.));
#86178=CARTESIAN_POINT('Ctrl Pts',(455.401407401473,27.0741275496278,27.0741275496278));
#86179=CARTESIAN_POINT('Ctrl Pts',(455.401407401473,0.,27.0741275496278));
#86180=CARTESIAN_POINT('Ctrl Pts',(455.401407401473,-27.0741275496278,27.0741275496278));
#86181=CARTESIAN_POINT('Ctrl Pts',(455.401407401473,-27.0741275496278,0.));
#86182=CARTESIAN_POINT('Ctrl Pts',(455.401407401473,-27.0741275496278,-27.0741275496278));
#86183=CARTESIAN_POINT('Ctrl Pts',(455.401407401473,0.,-27.0741275496278));
#86184=CARTESIAN_POINT('Ctrl Pts',(455.401407401473,27.0741275496278,-27.0741275496278));
#86185=CARTESIAN_POINT('Ctrl Pts',(455.401407401473,27.0741275496278,0.));
#86186=CARTESIAN_POINT('Ctrl Pts',(455.965472189203,26.4565068762911,0.));
#86187=CARTESIAN_POINT('Ctrl Pts',(455.965472189203,26.456506876291,26.456506876291));
#86188=CARTESIAN_POINT('Ctrl Pts',(455.965472189203,0.,26.4565068762911));
#86189=CARTESIAN_POINT('Ctrl Pts',(455.965472189203,-26.456506876291,26.456506876291));
#86190=CARTESIAN_POINT('Ctrl Pts',(455.965472189203,-26.4565068762911,0.));
#86191=CARTESIAN_POINT('Ctrl Pts',(455.965472189203,-26.456506876291,-26.456506876291));
#86192=CARTESIAN_POINT('Ctrl Pts',(455.965472189203,0.,-26.4565068762911));
#86193=CARTESIAN_POINT('Ctrl Pts',(455.965472189203,26.456506876291,-26.456506876291));
#86194=CARTESIAN_POINT('Ctrl Pts',(455.965472189203,26.4565068762911,0.));
#86195=CARTESIAN_POINT('Ctrl Pts',(456.499992138814,25.6788942561824,0.));
#86196=CARTESIAN_POINT('Ctrl Pts',(456.499992138814,25.6788942561824,25.6788942561824));
#86197=CARTESIAN_POINT('Ctrl Pts',(456.499992138814,0.,25.6788942561824));
#86198=CARTESIAN_POINT('Ctrl Pts',(456.499992138814,-25.6788942561824,25.6788942561824));
#86199=CARTESIAN_POINT('Ctrl Pts',(456.499992138814,-25.6788942561824,0.));
#86200=CARTESIAN_POINT('Ctrl Pts',(456.499992138814,-25.6788942561824,-25.6788942561824));
#86201=CARTESIAN_POINT('Ctrl Pts',(456.499992138814,0.,-25.6788942561824));
#86202=CARTESIAN_POINT('Ctrl Pts',(456.499992138814,25.6788942561824,-25.6788942561824));
#86203=CARTESIAN_POINT('Ctrl Pts',(456.499992138814,25.6788942561824,0.));
#86204=CARTESIAN_POINT('Ctrl Pts',(457.035460070478,24.8175654564571,0.));
#86205=CARTESIAN_POINT('Ctrl Pts',(457.035460070478,24.8175654564571,24.8175654564571));
#86206=CARTESIAN_POINT('Ctrl Pts',(457.035460070478,0.,24.8175654564571));
#86207=CARTESIAN_POINT('Ctrl Pts',(457.035460070478,-24.8175654564571,24.8175654564571));
#86208=CARTESIAN_POINT('Ctrl Pts',(457.035460070478,-24.8175654564571,0.));
#86209=CARTESIAN_POINT('Ctrl Pts',(457.035460070478,-24.8175654564571,-24.8175654564571));
#86210=CARTESIAN_POINT('Ctrl Pts',(457.035460070478,0.,-24.8175654564571));
#86211=CARTESIAN_POINT('Ctrl Pts',(457.035460070478,24.8175654564571,-24.8175654564571));
#86212=CARTESIAN_POINT('Ctrl Pts',(457.035460070478,24.8175654564571,0.));
#86213=CARTESIAN_POINT('Ctrl Pts',(457.601703267487,23.960894022917,0.));
#86214=CARTESIAN_POINT('Ctrl Pts',(457.601703267487,23.960894022917,23.960894022917));
#86215=CARTESIAN_POINT('Ctrl Pts',(457.601703267487,0.,23.960894022917));
#86216=CARTESIAN_POINT('Ctrl Pts',(457.601703267487,-23.960894022917,23.960894022917));
#86217=CARTESIAN_POINT('Ctrl Pts',(457.601703267487,-23.960894022917,0.));
#86218=CARTESIAN_POINT('Ctrl Pts',(457.601703267487,-23.960894022917,-23.960894022917));
#86219=CARTESIAN_POINT('Ctrl Pts',(457.601703267487,0.,-23.960894022917));
#86220=CARTESIAN_POINT('Ctrl Pts',(457.601703267487,23.960894022917,-23.960894022917));
#86221=CARTESIAN_POINT('Ctrl Pts',(457.601703267487,23.960894022917,0.));
#86222=CARTESIAN_POINT('Ctrl Pts',(458.220427115088,23.1990940255842,0.));
#86223=CARTESIAN_POINT('Ctrl Pts',(458.220427115088,23.1990940255842,23.1990940255842));
#86224=CARTESIAN_POINT('Ctrl Pts',(458.220427115088,0.,23.1990940255842));
#86225=CARTESIAN_POINT('Ctrl Pts',(458.220427115088,-23.1990940255842,23.1990940255842));
#86226=CARTESIAN_POINT('Ctrl Pts',(458.220427115088,-23.1990940255842,0.));
#86227=CARTESIAN_POINT('Ctrl Pts',(458.220427115088,-23.1990940255842,-23.1990940255842));
#86228=CARTESIAN_POINT('Ctrl Pts',(458.220427115088,0.,-23.1990940255842));
#86229=CARTESIAN_POINT('Ctrl Pts',(458.220427115088,23.1990940255842,-23.1990940255842));
#86230=CARTESIAN_POINT('Ctrl Pts',(458.220427115088,23.1990940255842,0.));
#86231=CARTESIAN_POINT('Ctrl Pts',(458.89594022623,22.6137057693112,0.));
#86232=CARTESIAN_POINT('Ctrl Pts',(458.89594022623,22.6137057693112,22.6137057693112));
#86233=CARTESIAN_POINT('Ctrl Pts',(458.89594022623,0.,22.6137057693112));
#86234=CARTESIAN_POINT('Ctrl Pts',(458.89594022623,-22.6137057693112,22.6137057693112));
#86235=CARTESIAN_POINT('Ctrl Pts',(458.89594022623,-22.6137057693112,0.));
#86236=CARTESIAN_POINT('Ctrl Pts',(458.89594022623,-22.6137057693112,-22.6137057693112));
#86237=CARTESIAN_POINT('Ctrl Pts',(458.89594022623,0.,-22.6137057693112));
#86238=CARTESIAN_POINT('Ctrl Pts',(458.89594022623,22.6137057693112,-22.6137057693112));
#86239=CARTESIAN_POINT('Ctrl Pts',(458.89594022623,22.6137057693112,0.));
#86240=CARTESIAN_POINT('Ctrl Pts',(459.612787385745,22.2695103984714,0.));
#86241=CARTESIAN_POINT('Ctrl Pts',(459.612787385745,22.2695103984714,22.2695103984714));
#86242=CARTESIAN_POINT('Ctrl Pts',(459.612787385745,0.,22.2695103984714));
#86243=CARTESIAN_POINT('Ctrl Pts',(459.612787385745,-22.2695103984714,22.2695103984714));
#86244=CARTESIAN_POINT('Ctrl Pts',(459.612787385745,-22.2695103984714,0.));
#86245=CARTESIAN_POINT('Ctrl Pts',(459.612787385745,-22.2695103984714,-22.2695103984714));
#86246=CARTESIAN_POINT('Ctrl Pts',(459.612787385745,0.,-22.2695103984714));
#86247=CARTESIAN_POINT('Ctrl Pts',(459.612787385745,22.2695103984714,-22.2695103984714));
#86248=CARTESIAN_POINT('Ctrl Pts',(459.612787385745,22.2695103984714,0.));
#86249=CARTESIAN_POINT('Ctrl Pts',(460.34599973061,22.211124033265,0.));
#86250=CARTESIAN_POINT('Ctrl Pts',(460.34599973061,22.211124033265,22.211124033265));
#86251=CARTESIAN_POINT('Ctrl Pts',(460.34599973061,0.,22.211124033265));
#86252=CARTESIAN_POINT('Ctrl Pts',(460.34599973061,-22.211124033265,22.211124033265));
#86253=CARTESIAN_POINT('Ctrl Pts',(460.34599973061,-22.211124033265,0.));
#86254=CARTESIAN_POINT('Ctrl Pts',(460.34599973061,-22.211124033265,-22.211124033265));
#86255=CARTESIAN_POINT('Ctrl Pts',(460.34599973061,0.,-22.211124033265));
#86256=CARTESIAN_POINT('Ctrl Pts',(460.34599973061,22.211124033265,-22.211124033265));
#86257=CARTESIAN_POINT('Ctrl Pts',(460.34599973061,22.211124033265,0.));
#86258=CARTESIAN_POINT('Ctrl Pts',(461.068363394086,22.4586715684347,0.));
#86259=CARTESIAN_POINT('Ctrl Pts',(461.068363394086,22.4586715684347,22.4586715684347));
#86260=CARTESIAN_POINT('Ctrl Pts',(461.068363394086,0.,22.4586715684347));
#86261=CARTESIAN_POINT('Ctrl Pts',(461.068363394086,-22.4586715684347,22.4586715684347));
#86262=CARTESIAN_POINT('Ctrl Pts',(461.068363394086,-22.4586715684347,0.));
#86263=CARTESIAN_POINT('Ctrl Pts',(461.068363394086,-22.4586715684347,-22.4586715684347));
#86264=CARTESIAN_POINT('Ctrl Pts',(461.068363394086,0.,-22.4586715684347));
#86265=CARTESIAN_POINT('Ctrl Pts',(461.068363394086,22.4586715684347,-22.4586715684347));
#86266=CARTESIAN_POINT('Ctrl Pts',(461.068363394086,22.4586715684347,0.));
#86267=CARTESIAN_POINT('Ctrl Pts',(461.759168926054,23.0034635988083,0.));
#86268=CARTESIAN_POINT('Ctrl Pts',(461.759168926054,23.0034635988083,23.0034635988083));
#86269=CARTESIAN_POINT('Ctrl Pts',(461.759168926054,0.,23.0034635988083));
#86270=CARTESIAN_POINT('Ctrl Pts',(461.759168926054,-23.0034635988083,23.0034635988083));
#86271=CARTESIAN_POINT('Ctrl Pts',(461.759168926054,-23.0034635988083,0.));
#86272=CARTESIAN_POINT('Ctrl Pts',(461.759168926054,-23.0034635988083,-23.0034635988083));
#86273=CARTESIAN_POINT('Ctrl Pts',(461.759168926054,0.,-23.0034635988083));
#86274=CARTESIAN_POINT('Ctrl Pts',(461.759168926054,23.0034635988083,-23.0034635988083));
#86275=CARTESIAN_POINT('Ctrl Pts',(461.759168926054,23.0034635988083,0.));
#86276=CARTESIAN_POINT('Ctrl Pts',(462.411522978371,23.8046505711925,0.));
#86277=CARTESIAN_POINT('Ctrl Pts',(462.411522978371,23.8046505711925,23.8046505711925));
#86278=CARTESIAN_POINT('Ctrl Pts',(462.411522978371,0.,23.8046505711925));
#86279=CARTESIAN_POINT('Ctrl Pts',(462.411522978371,-23.8046505711925,23.8046505711925));
#86280=CARTESIAN_POINT('Ctrl Pts',(462.411522978371,-23.8046505711925,0.));
#86281=CARTESIAN_POINT('Ctrl Pts',(462.411522978371,-23.8046505711925,-23.8046505711925));
#86282=CARTESIAN_POINT('Ctrl Pts',(462.411522978371,0.,-23.8046505711925));
#86283=CARTESIAN_POINT('Ctrl Pts',(462.411522978371,23.8046505711925,-23.8046505711925));
#86284=CARTESIAN_POINT('Ctrl Pts',(462.411522978371,23.8046505711925,0.));
#86285=CARTESIAN_POINT('Ctrl Pts',(463.028833596255,24.7993805174891,0.));
#86286=CARTESIAN_POINT('Ctrl Pts',(463.028833596255,24.7993805174891,24.7993805174891));
#86287=CARTESIAN_POINT('Ctrl Pts',(463.028833596255,0.,24.7993805174891));
#86288=CARTESIAN_POINT('Ctrl Pts',(463.028833596255,-24.7993805174891,24.7993805174891));
#86289=CARTESIAN_POINT('Ctrl Pts',(463.028833596255,-24.7993805174891,0.));
#86290=CARTESIAN_POINT('Ctrl Pts',(463.028833596255,-24.7993805174891,-24.7993805174891));
#86291=CARTESIAN_POINT('Ctrl Pts',(463.028833596255,0.,-24.7993805174891));
#86292=CARTESIAN_POINT('Ctrl Pts',(463.028833596255,24.7993805174891,-24.7993805174891));
#86293=CARTESIAN_POINT('Ctrl Pts',(463.028833596255,24.7993805174891,0.));
#86294=CARTESIAN_POINT('Ctrl Pts',(463.621964437201,25.9120692248671,0.));
#86295=CARTESIAN_POINT('Ctrl Pts',(463.621964437201,25.9120692248671,25.9120692248671));
#86296=CARTESIAN_POINT('Ctrl Pts',(463.621964437201,0.,25.9120692248671));
#86297=CARTESIAN_POINT('Ctrl Pts',(463.621964437201,-25.9120692248671,25.9120692248671));
#86298=CARTESIAN_POINT('Ctrl Pts',(463.621964437201,-25.9120692248671,0.));
#86299=CARTESIAN_POINT('Ctrl Pts',(463.621964437201,-25.9120692248671,-25.9120692248671));
#86300=CARTESIAN_POINT('Ctrl Pts',(463.621964437201,0.,-25.9120692248671));
#86301=CARTESIAN_POINT('Ctrl Pts',(463.621964437201,25.9120692248671,-25.9120692248671));
#86302=CARTESIAN_POINT('Ctrl Pts',(463.621964437201,25.9120692248671,0.));
#86303=CARTESIAN_POINT('Ctrl Pts',(464.206176993335,27.0638091657224,0.));
#86304=CARTESIAN_POINT('Ctrl Pts',(464.206176993335,27.0638091657224,27.0638091657224));
#86305=CARTESIAN_POINT('Ctrl Pts',(464.206176993335,0.,27.0638091657224));
#86306=CARTESIAN_POINT('Ctrl Pts',(464.206176993335,-27.0638091657224,27.0638091657224));
#86307=CARTESIAN_POINT('Ctrl Pts',(464.206176993335,-27.0638091657224,0.));
#86308=CARTESIAN_POINT('Ctrl Pts',(464.206176993335,-27.0638091657224,-27.0638091657224));
#86309=CARTESIAN_POINT('Ctrl Pts',(464.206176993335,0.,-27.0638091657224));
#86310=CARTESIAN_POINT('Ctrl Pts',(464.206176993335,27.0638091657224,-27.0638091657224));
#86311=CARTESIAN_POINT('Ctrl Pts',(464.206176993335,27.0638091657224,0.));
#86312=CARTESIAN_POINT('Ctrl Pts',(464.798092368276,28.1821479594276,0.));
#86313=CARTESIAN_POINT('Ctrl Pts',(464.798092368276,28.1821479594276,28.1821479594276));
#86314=CARTESIAN_POINT('Ctrl Pts',(464.798092368276,0.,28.1821479594276));
#86315=CARTESIAN_POINT('Ctrl Pts',(464.798092368276,-28.1821479594276,28.1821479594276));
#86316=CARTESIAN_POINT('Ctrl Pts',(464.798092368276,-28.1821479594276,0.));
#86317=CARTESIAN_POINT('Ctrl Pts',(464.798092368276,-28.1821479594276,-28.1821479594276));
#86318=CARTESIAN_POINT('Ctrl Pts',(464.798092368276,0.,-28.1821479594276));
#86319=CARTESIAN_POINT('Ctrl Pts',(464.798092368276,28.1821479594276,-28.1821479594276));
#86320=CARTESIAN_POINT('Ctrl Pts',(464.798092368276,28.1821479594276,0.));
#86321=CARTESIAN_POINT('Ctrl Pts',(465.412818401399,29.2096983338665,0.));
#86322=CARTESIAN_POINT('Ctrl Pts',(465.412818401399,29.2096983338665,29.2096983338665));
#86323=CARTESIAN_POINT('Ctrl Pts',(465.412818401399,0.,29.2096983338665));
#86324=CARTESIAN_POINT('Ctrl Pts',(465.412818401399,-29.2096983338665,29.2096983338665));
#86325=CARTESIAN_POINT('Ctrl Pts',(465.412818401399,-29.2096983338665,0.));
#86326=CARTESIAN_POINT('Ctrl Pts',(465.412818401399,-29.2096983338665,-29.2096983338665));
#86327=CARTESIAN_POINT('Ctrl Pts',(465.412818401399,0.,-29.2096983338665));
#86328=CARTESIAN_POINT('Ctrl Pts',(465.412818401399,29.2096983338665,-29.2096983338665));
#86329=CARTESIAN_POINT('Ctrl Pts',(465.412818401399,29.2096983338665,0.));
#86330=CARTESIAN_POINT('Ctrl Pts',(466.060566868545,30.1158330796105,0.));
#86331=CARTESIAN_POINT('Ctrl Pts',(466.060566868545,30.1158330796105,30.1158330796105));
#86332=CARTESIAN_POINT('Ctrl Pts',(466.060566868545,0.,30.1158330796105));
#86333=CARTESIAN_POINT('Ctrl Pts',(466.060566868545,-30.1158330796105,30.1158330796105));
#86334=CARTESIAN_POINT('Ctrl Pts',(466.060566868545,-30.1158330796105,0.));
#86335=CARTESIAN_POINT('Ctrl Pts',(466.060566868545,-30.1158330796105,-30.1158330796105));
#86336=CARTESIAN_POINT('Ctrl Pts',(466.060566868545,0.,-30.1158330796105));
#86337=CARTESIAN_POINT('Ctrl Pts',(466.060566868545,30.1158330796105,-30.1158330796105));
#86338=CARTESIAN_POINT('Ctrl Pts',(466.060566868545,30.1158330796105,0.));
#86339=CARTESIAN_POINT('Ctrl Pts',(466.745838674916,30.8932609419353,0.));
#86340=CARTESIAN_POINT('Ctrl Pts',(466.745838674916,30.8932609419353,30.8932609419353));
#86341=CARTESIAN_POINT('Ctrl Pts',(466.745838674916,0.,30.8932609419353));
#86342=CARTESIAN_POINT('Ctrl Pts',(466.745838674916,-30.8932609419353,30.8932609419353));
#86343=CARTESIAN_POINT('Ctrl Pts',(466.745838674916,-30.8932609419353,0.));
#86344=CARTESIAN_POINT('Ctrl Pts',(466.745838674916,-30.8932609419353,-30.8932609419353));
#86345=CARTESIAN_POINT('Ctrl Pts',(466.745838674916,0.,-30.8932609419353));
#86346=CARTESIAN_POINT('Ctrl Pts',(466.745838674916,30.8932609419353,-30.8932609419353));
#86347=CARTESIAN_POINT('Ctrl Pts',(466.745838674916,30.8932609419353,0.));
#86348=CARTESIAN_POINT('Ctrl Pts',(467.467796162958,31.5476428728425,0.));
#86349=CARTESIAN_POINT('Ctrl Pts',(467.467796162958,31.5476428728425,31.5476428728425));
#86350=CARTESIAN_POINT('Ctrl Pts',(467.467796162958,0.,31.5476428728425));
#86351=CARTESIAN_POINT('Ctrl Pts',(467.467796162958,-31.5476428728425,31.5476428728425));
#86352=CARTESIAN_POINT('Ctrl Pts',(467.467796162958,-31.5476428728425,0.));
#86353=CARTESIAN_POINT('Ctrl Pts',(467.467796162958,-31.5476428728425,-31.5476428728425));
#86354=CARTESIAN_POINT('Ctrl Pts',(467.467796162958,0.,-31.5476428728425));
#86355=CARTESIAN_POINT('Ctrl Pts',(467.467796162958,31.5476428728425,-31.5476428728425));
#86356=CARTESIAN_POINT('Ctrl Pts',(467.467796162958,31.5476428728425,0.));
#86357=CARTESIAN_POINT('Ctrl Pts',(468.220253767095,32.0894344364089,0.));
#86358=CARTESIAN_POINT('Ctrl Pts',(468.220253767095,32.0894344364089,32.0894344364089));
#86359=CARTESIAN_POINT('Ctrl Pts',(468.220253767095,0.,32.0894344364089));
#86360=CARTESIAN_POINT('Ctrl Pts',(468.220253767095,-32.0894344364089,32.0894344364089));
#86361=CARTESIAN_POINT('Ctrl Pts',(468.220253767095,-32.0894344364089,0.));
#86362=CARTESIAN_POINT('Ctrl Pts',(468.220253767095,-32.0894344364089,-32.0894344364089));
#86363=CARTESIAN_POINT('Ctrl Pts',(468.220253767095,0.,-32.0894344364089));
#86364=CARTESIAN_POINT('Ctrl Pts',(468.220253767095,32.0894344364089,-32.0894344364089));
#86365=CARTESIAN_POINT('Ctrl Pts',(468.220253767095,32.0894344364089,0.));
#86366=CARTESIAN_POINT('Ctrl Pts',(468.991825973097,32.5247950832038,0.));
#86367=CARTESIAN_POINT('Ctrl Pts',(468.991825973097,32.5247950832038,32.5247950832038));
#86368=CARTESIAN_POINT('Ctrl Pts',(468.991825973097,0.,32.5247950832038));
#86369=CARTESIAN_POINT('Ctrl Pts',(468.991825973097,-32.5247950832038,32.5247950832038));
#86370=CARTESIAN_POINT('Ctrl Pts',(468.991825973097,-32.5247950832038,0.));
#86371=CARTESIAN_POINT('Ctrl Pts',(468.991825973097,-32.5247950832038,-32.5247950832038));
#86372=CARTESIAN_POINT('Ctrl Pts',(468.991825973097,0.,-32.5247950832038));
#86373=CARTESIAN_POINT('Ctrl Pts',(468.991825973097,32.5247950832038,-32.5247950832038));
#86374=CARTESIAN_POINT('Ctrl Pts',(468.991825973097,32.5247950832038,0.));
#86375=CARTESIAN_POINT('Ctrl Pts',(469.766000094273,32.8469261327295,0.));
#86376=CARTESIAN_POINT('Ctrl Pts',(469.766000094273,32.8469261327295,32.8469261327295));
#86377=CARTESIAN_POINT('Ctrl Pts',(469.766000094273,0.,32.8469261327295));
#86378=CARTESIAN_POINT('Ctrl Pts',(469.766000094273,-32.8469261327295,32.8469261327295));
#86379=CARTESIAN_POINT('Ctrl Pts',(469.766000094273,-32.8469261327295,0.));
#86380=CARTESIAN_POINT('Ctrl Pts',(469.766000094273,-32.8469261327295,-32.8469261327295));
#86381=CARTESIAN_POINT('Ctrl Pts',(469.766000094273,0.,-32.8469261327295));
#86382=CARTESIAN_POINT('Ctrl Pts',(469.766000094273,32.8469261327295,-32.8469261327295));
#86383=CARTESIAN_POINT('Ctrl Pts',(469.766000094273,32.8469261327295,0.));
#86384=CARTESIAN_POINT('Ctrl Pts',(470.521241805588,33.0271235924796,0.));
#86385=CARTESIAN_POINT('Ctrl Pts',(470.521241805588,33.0271235924796,33.0271235924796));
#86386=CARTESIAN_POINT('Ctrl Pts',(470.521241805588,0.,33.0271235924796));
#86387=CARTESIAN_POINT('Ctrl Pts',(470.521241805588,-33.0271235924796,33.0271235924796));
#86388=CARTESIAN_POINT('Ctrl Pts',(470.521241805588,-33.0271235924796,0.));
#86389=CARTESIAN_POINT('Ctrl Pts',(470.521241805588,-33.0271235924796,-33.0271235924796));
#86390=CARTESIAN_POINT('Ctrl Pts',(470.521241805588,0.,-33.0271235924796));
#86391=CARTESIAN_POINT('Ctrl Pts',(470.521241805588,33.0271235924796,-33.0271235924796));
#86392=CARTESIAN_POINT('Ctrl Pts',(470.521241805588,33.0271235924796,0.));
#86393=CARTESIAN_POINT('Ctrl Pts',(471.236383616488,33.0283632061197,0.));
#86394=CARTESIAN_POINT('Ctrl Pts',(471.236383616488,33.0283632061197,33.0283632061197));
#86395=CARTESIAN_POINT('Ctrl Pts',(471.236383616488,0.,33.0283632061197));
#86396=CARTESIAN_POINT('Ctrl Pts',(471.236383616488,-33.0283632061197,33.0283632061197));
#86397=CARTESIAN_POINT('Ctrl Pts',(471.236383616488,-33.0283632061197,0.));
#86398=CARTESIAN_POINT('Ctrl Pts',(471.236383616488,-33.0283632061197,-33.0283632061197));
#86399=CARTESIAN_POINT('Ctrl Pts',(471.236383616488,0.,-33.0283632061197));
#86400=CARTESIAN_POINT('Ctrl Pts',(471.236383616488,33.0283632061197,-33.0283632061197));
#86401=CARTESIAN_POINT('Ctrl Pts',(471.236383616488,33.0283632061197,0.));
#86402=CARTESIAN_POINT('Ctrl Pts',(471.89635548407,32.8195310910232,0.));
#86403=CARTESIAN_POINT('Ctrl Pts',(471.89635548407,32.8195310910232,32.8195310910232));
#86404=CARTESIAN_POINT('Ctrl Pts',(471.89635548407,0.,32.8195310910232));
#86405=CARTESIAN_POINT('Ctrl Pts',(471.89635548407,-32.8195310910232,32.8195310910232));
#86406=CARTESIAN_POINT('Ctrl Pts',(471.89635548407,-32.8195310910232,0.));
#86407=CARTESIAN_POINT('Ctrl Pts',(471.89635548407,-32.8195310910232,-32.8195310910232));
#86408=CARTESIAN_POINT('Ctrl Pts',(471.89635548407,0.,-32.8195310910232));
#86409=CARTESIAN_POINT('Ctrl Pts',(471.89635548407,32.8195310910232,-32.8195310910232));
#86410=CARTESIAN_POINT('Ctrl Pts',(471.89635548407,32.8195310910232,0.));
#86411=CARTESIAN_POINT('Ctrl Pts',(472.497221742613,32.388473647408,0.));
#86412=CARTESIAN_POINT('Ctrl Pts',(472.497221742613,32.388473647408,32.388473647408));
#86413=CARTESIAN_POINT('Ctrl Pts',(472.497221742613,0.,32.388473647408));
#86414=CARTESIAN_POINT('Ctrl Pts',(472.497221742613,-32.388473647408,32.388473647408));
#86415=CARTESIAN_POINT('Ctrl Pts',(472.497221742613,-32.388473647408,0.));
#86416=CARTESIAN_POINT('Ctrl Pts',(472.497221742613,-32.388473647408,-32.388473647408));
#86417=CARTESIAN_POINT('Ctrl Pts',(472.497221742613,0.,-32.388473647408));
#86418=CARTESIAN_POINT('Ctrl Pts',(472.497221742613,32.388473647408,-32.388473647408));
#86419=CARTESIAN_POINT('Ctrl Pts',(472.497221742613,32.388473647408,0.));
#86420=CARTESIAN_POINT('Ctrl Pts',(473.052965117723,31.7579657390958,0.));
#86421=CARTESIAN_POINT('Ctrl Pts',(473.052965117723,31.7579657390958,31.7579657390958));
#86422=CARTESIAN_POINT('Ctrl Pts',(473.052965117723,0.,31.7579657390958));
#86423=CARTESIAN_POINT('Ctrl Pts',(473.052965117723,-31.7579657390958,31.7579657390958));
#86424=CARTESIAN_POINT('Ctrl Pts',(473.052965117723,-31.7579657390958,0.));
#86425=CARTESIAN_POINT('Ctrl Pts',(473.052965117723,-31.7579657390958,-31.7579657390958));
#86426=CARTESIAN_POINT('Ctrl Pts',(473.052965117723,0.,-31.7579657390958));
#86427=CARTESIAN_POINT('Ctrl Pts',(473.052965117723,31.7579657390958,-31.7579657390958));
#86428=CARTESIAN_POINT('Ctrl Pts',(473.052965117723,31.7579657390958,0.));
#86429=CARTESIAN_POINT('Ctrl Pts',(473.589859436769,30.9807114425168,0.));
#86430=CARTESIAN_POINT('Ctrl Pts',(473.589859436769,30.9807114425168,30.9807114425168));
#86431=CARTESIAN_POINT('Ctrl Pts',(473.589859436769,0.,30.9807114425168));
#86432=CARTESIAN_POINT('Ctrl Pts',(473.589859436769,-30.9807114425168,30.9807114425168));
#86433=CARTESIAN_POINT('Ctrl Pts',(473.589859436769,-30.9807114425168,0.));
#86434=CARTESIAN_POINT('Ctrl Pts',(473.589859436769,-30.9807114425168,-30.9807114425168));
#86435=CARTESIAN_POINT('Ctrl Pts',(473.589859436769,0.,-30.9807114425168));
#86436=CARTESIAN_POINT('Ctrl Pts',(473.589859436769,30.9807114425168,-30.9807114425168));
#86437=CARTESIAN_POINT('Ctrl Pts',(473.589859436769,30.9807114425168,0.));
#86438=CARTESIAN_POINT('Ctrl Pts',(474.138366833956,30.1297846394355,0.));
#86439=CARTESIAN_POINT('Ctrl Pts',(474.138366833956,30.1297846394355,30.1297846394355));
#86440=CARTESIAN_POINT('Ctrl Pts',(474.138366833956,0.,30.1297846394355));
#86441=CARTESIAN_POINT('Ctrl Pts',(474.138366833956,-30.1297846394355,30.1297846394355));
#86442=CARTESIAN_POINT('Ctrl Pts',(474.138366833956,-30.1297846394355,0.));
#86443=CARTESIAN_POINT('Ctrl Pts',(474.138366833956,-30.1297846394355,-30.1297846394355));
#86444=CARTESIAN_POINT('Ctrl Pts',(474.138366833956,0.,-30.1297846394355));
#86445=CARTESIAN_POINT('Ctrl Pts',(474.138366833956,30.1297846394355,-30.1297846394355));
#86446=CARTESIAN_POINT('Ctrl Pts',(474.138366833956,30.1297846394355,0.));
#86447=CARTESIAN_POINT('Ctrl Pts',(474.725466937653,29.2906333134204,0.));
#86448=CARTESIAN_POINT('Ctrl Pts',(474.725466937653,29.2906333134204,29.2906333134204));
#86449=CARTESIAN_POINT('Ctrl Pts',(474.725466937653,0.,29.2906333134204));
#86450=CARTESIAN_POINT('Ctrl Pts',(474.725466937653,-29.2906333134204,29.2906333134204));
#86451=CARTESIAN_POINT('Ctrl Pts',(474.725466937653,-29.2906333134204,0.));
#86452=CARTESIAN_POINT('Ctrl Pts',(474.725466937653,-29.2906333134204,-29.2906333134204));
#86453=CARTESIAN_POINT('Ctrl Pts',(474.725466937653,0.,-29.2906333134204));
#86454=CARTESIAN_POINT('Ctrl Pts',(474.725466937653,29.2906333134204,-29.2906333134204));
#86455=CARTESIAN_POINT('Ctrl Pts',(474.725466937653,29.2906333134204,0.));
#86456=CARTESIAN_POINT('Ctrl Pts',(475.36775535895,28.5524756034697,0.));
#86457=CARTESIAN_POINT('Ctrl Pts',(475.36775535895,28.5524756034697,28.5524756034697));
#86458=CARTESIAN_POINT('Ctrl Pts',(475.36775535895,0.,28.5524756034697));
#86459=CARTESIAN_POINT('Ctrl Pts',(475.36775535895,-28.5524756034697,28.5524756034697));
#86460=CARTESIAN_POINT('Ctrl Pts',(475.36775535895,-28.5524756034697,0.));
#86461=CARTESIAN_POINT('Ctrl Pts',(475.36775535895,-28.5524756034697,-28.5524756034697));
#86462=CARTESIAN_POINT('Ctrl Pts',(475.36775535895,0.,-28.5524756034697));
#86463=CARTESIAN_POINT('Ctrl Pts',(475.36775535895,28.5524756034697,-28.5524756034697));
#86464=CARTESIAN_POINT('Ctrl Pts',(475.36775535895,28.5524756034697,0.));
#86465=CARTESIAN_POINT('Ctrl Pts',(476.061833863912,27.999869975222,0.));
#86466=CARTESIAN_POINT('Ctrl Pts',(476.061833863912,27.999869975222,27.999869975222));
#86467=CARTESIAN_POINT('Ctrl Pts',(476.061833863912,0.,27.999869975222));
#86468=CARTESIAN_POINT('Ctrl Pts',(476.061833863912,-27.999869975222,27.999869975222));
#86469=CARTESIAN_POINT('Ctrl Pts',(476.061833863912,-27.999869975222,0.));
#86470=CARTESIAN_POINT('Ctrl Pts',(476.061833863912,-27.999869975222,-27.999869975222));
#86471=CARTESIAN_POINT('Ctrl Pts',(476.061833863912,0.,-27.999869975222));
#86472=CARTESIAN_POINT('Ctrl Pts',(476.061833863912,27.999869975222,-27.999869975222));
#86473=CARTESIAN_POINT('Ctrl Pts',(476.061833863912,27.999869975222,0.));
#86474=CARTESIAN_POINT('Ctrl Pts',(476.786527826342,27.7044708275784,0.));
#86475=CARTESIAN_POINT('Ctrl Pts',(476.786527826342,27.7044708275784,27.7044708275784));
#86476=CARTESIAN_POINT('Ctrl Pts',(476.786527826342,0.,27.7044708275784));
#86477=CARTESIAN_POINT('Ctrl Pts',(476.786527826342,-27.7044708275784,27.7044708275784));
#86478=CARTESIAN_POINT('Ctrl Pts',(476.786527826342,-27.7044708275784,0.));
#86479=CARTESIAN_POINT('Ctrl Pts',(476.786527826342,-27.7044708275784,-27.7044708275784));
#86480=CARTESIAN_POINT('Ctrl Pts',(476.786527826342,0.,-27.7044708275784));
#86481=CARTESIAN_POINT('Ctrl Pts',(476.786527826342,27.7044708275784,-27.7044708275784));
#86482=CARTESIAN_POINT('Ctrl Pts',(476.786527826342,27.7044708275784,0.));
#86483=CARTESIAN_POINT('Ctrl Pts',(477.513843400759,27.7164651257201,0.));
#86484=CARTESIAN_POINT('Ctrl Pts',(477.513843400759,27.7164651257201,27.7164651257201));
#86485=CARTESIAN_POINT('Ctrl Pts',(477.513843400759,0.,27.7164651257201));
#86486=CARTESIAN_POINT('Ctrl Pts',(477.513843400759,-27.7164651257201,27.7164651257201));
#86487=CARTESIAN_POINT('Ctrl Pts',(477.513843400759,-27.7164651257201,0.));
#86488=CARTESIAN_POINT('Ctrl Pts',(477.513843400759,-27.7164651257201,-27.7164651257201));
#86489=CARTESIAN_POINT('Ctrl Pts',(477.513843400759,0.,-27.7164651257201));
#86490=CARTESIAN_POINT('Ctrl Pts',(477.513843400759,27.7164651257201,-27.7164651257201));
#86491=CARTESIAN_POINT('Ctrl Pts',(477.513843400759,27.7164651257201,0.));
#86492=CARTESIAN_POINT('Ctrl Pts',(478.216787070683,28.0569960770463,0.));
#86493=CARTESIAN_POINT('Ctrl Pts',(478.216787070683,28.0569960770463,28.0569960770463));
#86494=CARTESIAN_POINT('Ctrl Pts',(478.216787070683,0.,28.0569960770463));
#86495=CARTESIAN_POINT('Ctrl Pts',(478.216787070683,-28.0569960770463,28.0569960770463));
#86496=CARTESIAN_POINT('Ctrl Pts',(478.216787070683,-28.0569960770463,0.));
#86497=CARTESIAN_POINT('Ctrl Pts',(478.216787070683,-28.0569960770463,-28.0569960770463));
#86498=CARTESIAN_POINT('Ctrl Pts',(478.216787070683,0.,-28.0569960770463));
#86499=CARTESIAN_POINT('Ctrl Pts',(478.216787070683,28.0569960770463,-28.0569960770463));
#86500=CARTESIAN_POINT('Ctrl Pts',(478.216787070683,28.0569960770463,0.));
#86501=CARTESIAN_POINT('Ctrl Pts',(478.879732236756,28.7080878516033,0.));
#86502=CARTESIAN_POINT('Ctrl Pts',(478.879732236756,28.7080878516033,28.7080878516033));
#86503=CARTESIAN_POINT('Ctrl Pts',(478.879732236756,0.,28.7080878516033));
#86504=CARTESIAN_POINT('Ctrl Pts',(478.879732236756,-28.7080878516033,28.7080878516033));
#86505=CARTESIAN_POINT('Ctrl Pts',(478.879732236756,-28.7080878516033,0.));
#86506=CARTESIAN_POINT('Ctrl Pts',(478.879732236756,-28.7080878516033,-28.7080878516033));
#86507=CARTESIAN_POINT('Ctrl Pts',(478.879732236756,0.,-28.7080878516033));
#86508=CARTESIAN_POINT('Ctrl Pts',(478.879732236756,28.7080878516033,-28.7080878516033));
#86509=CARTESIAN_POINT('Ctrl Pts',(478.879732236756,28.7080878516033,0.));
#86510=CARTESIAN_POINT('Ctrl Pts',(479.503653522459,29.6103104041391,0.));
#86511=CARTESIAN_POINT('Ctrl Pts',(479.503653522459,29.6103104041391,29.6103104041391));
#86512=CARTESIAN_POINT('Ctrl Pts',(479.503653522459,0.,29.6103104041391));
#86513=CARTESIAN_POINT('Ctrl Pts',(479.503653522459,-29.6103104041391,29.6103104041391));
#86514=CARTESIAN_POINT('Ctrl Pts',(479.503653522459,-29.6103104041391,0.));
#86515=CARTESIAN_POINT('Ctrl Pts',(479.503653522459,-29.6103104041391,-29.6103104041391));
#86516=CARTESIAN_POINT('Ctrl Pts',(479.503653522459,0.,-29.6103104041391));
#86517=CARTESIAN_POINT('Ctrl Pts',(479.503653522459,29.6103104041391,-29.6103104041391));
#86518=CARTESIAN_POINT('Ctrl Pts',(479.503653522459,29.6103104041391,0.));
#86519=CARTESIAN_POINT('Ctrl Pts',(480.100216291509,30.6791487158265,0.));
#86520=CARTESIAN_POINT('Ctrl Pts',(480.100216291509,30.6791487158265,30.6791487158265));
#86521=CARTESIAN_POINT('Ctrl Pts',(480.100216291509,0.,30.6791487158265));
#86522=CARTESIAN_POINT('Ctrl Pts',(480.100216291509,-30.6791487158265,30.6791487158265));
#86523=CARTESIAN_POINT('Ctrl Pts',(480.100216291509,-30.6791487158265,0.));
#86524=CARTESIAN_POINT('Ctrl Pts',(480.100216291509,-30.6791487158265,-30.6791487158265));
#86525=CARTESIAN_POINT('Ctrl Pts',(480.100216291509,0.,-30.6791487158265));
#86526=CARTESIAN_POINT('Ctrl Pts',(480.100216291509,30.6791487158265,-30.6791487158265));
#86527=CARTESIAN_POINT('Ctrl Pts',(480.100216291509,30.6791487158265,0.));
#86528=CARTESIAN_POINT('Ctrl Pts',(480.687988617522,31.8177751379128,0.));
#86529=CARTESIAN_POINT('Ctrl Pts',(480.687988617522,31.8177751379128,31.8177751379128));
#86530=CARTESIAN_POINT('Ctrl Pts',(480.687988617522,0.,31.8177751379128));
#86531=CARTESIAN_POINT('Ctrl Pts',(480.687988617522,-31.8177751379128,31.8177751379128));
#86532=CARTESIAN_POINT('Ctrl Pts',(480.687988617522,-31.8177751379128,0.));
#86533=CARTESIAN_POINT('Ctrl Pts',(480.687988617522,-31.8177751379128,-31.8177751379128));
#86534=CARTESIAN_POINT('Ctrl Pts',(480.687988617522,0.,-31.8177751379128));
#86535=CARTESIAN_POINT('Ctrl Pts',(480.687988617522,31.8177751379128,-31.8177751379128));
#86536=CARTESIAN_POINT('Ctrl Pts',(480.687988617522,31.8177751379128,0.));
#86537=CARTESIAN_POINT('Ctrl Pts',(481.287852379122,32.9310860845041,0.));
#86538=CARTESIAN_POINT('Ctrl Pts',(481.287852379122,32.9310860845041,32.9310860845041));
#86539=CARTESIAN_POINT('Ctrl Pts',(481.287852379122,0.,32.9310860845041));
#86540=CARTESIAN_POINT('Ctrl Pts',(481.287852379122,-32.9310860845041,32.9310860845041));
#86541=CARTESIAN_POINT('Ctrl Pts',(481.287852379122,-32.9310860845041,0.));
#86542=CARTESIAN_POINT('Ctrl Pts',(481.287852379122,-32.9310860845041,-32.9310860845041));
#86543=CARTESIAN_POINT('Ctrl Pts',(481.287852379122,0.,-32.9310860845041));
#86544=CARTESIAN_POINT('Ctrl Pts',(481.287852379122,32.9310860845041,-32.9310860845041));
#86545=CARTESIAN_POINT('Ctrl Pts',(481.287852379122,32.9310860845041,0.));
#86546=CARTESIAN_POINT('Ctrl Pts',(481.91867866565,33.939552026335,0.));
#86547=CARTESIAN_POINT('Ctrl Pts',(481.91867866565,33.939552026335,33.939552026335));
#86548=CARTESIAN_POINT('Ctrl Pts',(481.91867866565,0.,33.939552026335));
#86549=CARTESIAN_POINT('Ctrl Pts',(481.91867866565,-33.939552026335,33.939552026335));
#86550=CARTESIAN_POINT('Ctrl Pts',(481.91867866565,-33.939552026335,0.));
#86551=CARTESIAN_POINT('Ctrl Pts',(481.91867866565,-33.939552026335,-33.939552026335));
#86552=CARTESIAN_POINT('Ctrl Pts',(481.91867866565,0.,-33.939552026335));
#86553=CARTESIAN_POINT('Ctrl Pts',(481.91867866565,33.939552026335,-33.939552026335));
#86554=CARTESIAN_POINT('Ctrl Pts',(481.91867866565,33.939552026335,0.));
#86555=CARTESIAN_POINT('Ctrl Pts',(482.593077053267,34.7923200716526,0.));
#86556=CARTESIAN_POINT('Ctrl Pts',(482.593077053267,34.7923200716526,34.7923200716526));
#86557=CARTESIAN_POINT('Ctrl Pts',(482.593077053267,0.,34.7923200716526));
#86558=CARTESIAN_POINT('Ctrl Pts',(482.593077053267,-34.7923200716526,34.7923200716526));
#86559=CARTESIAN_POINT('Ctrl Pts',(482.593077053267,-34.7923200716526,0.));
#86560=CARTESIAN_POINT('Ctrl Pts',(482.593077053267,-34.7923200716526,-34.7923200716526));
#86561=CARTESIAN_POINT('Ctrl Pts',(482.593077053267,0.,-34.7923200716526));
#86562=CARTESIAN_POINT('Ctrl Pts',(482.593077053267,34.7923200716526,-34.7923200716526));
#86563=CARTESIAN_POINT('Ctrl Pts',(482.593077053267,34.7923200716526,0.));
#86564=CARTESIAN_POINT('Ctrl Pts',(483.312607050695,35.4828759962818,0.));
#86565=CARTESIAN_POINT('Ctrl Pts',(483.312607050695,35.4828759962818,35.4828759962818));
#86566=CARTESIAN_POINT('Ctrl Pts',(483.312607050695,0.,35.4828759962818));
#86567=CARTESIAN_POINT('Ctrl Pts',(483.312607050695,-35.4828759962818,35.4828759962818));
#86568=CARTESIAN_POINT('Ctrl Pts',(483.312607050695,-35.4828759962818,0.));
#86569=CARTESIAN_POINT('Ctrl Pts',(483.312607050695,-35.4828759962818,-35.4828759962818));
#86570=CARTESIAN_POINT('Ctrl Pts',(483.312607050695,0.,-35.4828759962818));
#86571=CARTESIAN_POINT('Ctrl Pts',(483.312607050695,35.4828759962818,-35.4828759962818));
#86572=CARTESIAN_POINT('Ctrl Pts',(483.312607050695,35.4828759962818,0.));
#86573=CARTESIAN_POINT('Ctrl Pts',(484.06995894186,36.0346290589183,0.));
#86574=CARTESIAN_POINT('Ctrl Pts',(484.06995894186,36.0346290589183,36.0346290589183));
#86575=CARTESIAN_POINT('Ctrl Pts',(484.06995894186,0.,36.0346290589183));
#86576=CARTESIAN_POINT('Ctrl Pts',(484.06995894186,-36.0346290589183,36.0346290589183));
#86577=CARTESIAN_POINT('Ctrl Pts',(484.06995894186,-36.0346290589183,0.));
#86578=CARTESIAN_POINT('Ctrl Pts',(484.06995894186,-36.0346290589183,-36.0346290589183));
#86579=CARTESIAN_POINT('Ctrl Pts',(484.06995894186,0.,-36.0346290589183));
#86580=CARTESIAN_POINT('Ctrl Pts',(484.06995894186,36.0346290589183,-36.0346290589183));
#86581=CARTESIAN_POINT('Ctrl Pts',(484.06995894186,36.0346290589183,0.));
#86582=CARTESIAN_POINT('Ctrl Pts',(484.851896806652,36.4837434465982,0.));
#86583=CARTESIAN_POINT('Ctrl Pts',(484.851896806652,36.4837434465981,36.4837434465981));
#86584=CARTESIAN_POINT('Ctrl Pts',(484.851896806652,0.,36.4837434465982));
#86585=CARTESIAN_POINT('Ctrl Pts',(484.851896806652,-36.4837434465981,36.4837434465981));
#86586=CARTESIAN_POINT('Ctrl Pts',(484.851896806652,-36.4837434465982,0.));
#86587=CARTESIAN_POINT('Ctrl Pts',(484.851896806652,-36.4837434465981,-36.4837434465981));
#86588=CARTESIAN_POINT('Ctrl Pts',(484.851896806652,0.,-36.4837434465982));
#86589=CARTESIAN_POINT('Ctrl Pts',(484.851896806652,36.4837434465981,-36.4837434465981));
#86590=CARTESIAN_POINT('Ctrl Pts',(484.851896806652,36.4837434465982,0.));
#86591=CARTESIAN_POINT('Ctrl Pts',(485.641971156704,36.8618266029695,0.));
#86592=CARTESIAN_POINT('Ctrl Pts',(485.641971156704,36.8618266029695,36.8618266029695));
#86593=CARTESIAN_POINT('Ctrl Pts',(485.641971156704,0.,36.8618266029695));
#86594=CARTESIAN_POINT('Ctrl Pts',(485.641971156704,-36.8618266029695,36.8618266029695));
#86595=CARTESIAN_POINT('Ctrl Pts',(485.641971156704,-36.8618266029695,0.));
#86596=CARTESIAN_POINT('Ctrl Pts',(485.641971156704,-36.8618266029695,-36.8618266029695));
#86597=CARTESIAN_POINT('Ctrl Pts',(485.641971156704,0.,-36.8618266029695));
#86598=CARTESIAN_POINT('Ctrl Pts',(485.641971156704,36.8618266029695,-36.8618266029695));
#86599=CARTESIAN_POINT('Ctrl Pts',(485.641971156704,36.8618266029695,0.));
#86600=CARTESIAN_POINT('Ctrl Pts',(486.423221268854,37.1812508806874,0.));
#86601=CARTESIAN_POINT('Ctrl Pts',(486.423221268854,37.1812508806874,37.1812508806874));
#86602=CARTESIAN_POINT('Ctrl Pts',(486.423221268854,0.,37.1812508806874));
#86603=CARTESIAN_POINT('Ctrl Pts',(486.423221268854,-37.1812508806874,37.1812508806874));
#86604=CARTESIAN_POINT('Ctrl Pts',(486.423221268854,-37.1812508806874,0.));
#86605=CARTESIAN_POINT('Ctrl Pts',(486.423221268854,-37.1812508806874,-37.1812508806874));
#86606=CARTESIAN_POINT('Ctrl Pts',(486.423221268854,0.,-37.1812508806874));
#86607=CARTESIAN_POINT('Ctrl Pts',(486.423221268854,37.1812508806874,-37.1812508806874));
#86608=CARTESIAN_POINT('Ctrl Pts',(486.423221268854,37.1812508806874,0.));
#86609=CARTESIAN_POINT('Ctrl Pts',(487.181139377683,37.4129492363257,0.));
#86610=CARTESIAN_POINT('Ctrl Pts',(487.181139377683,37.4129492363257,37.4129492363257));
#86611=CARTESIAN_POINT('Ctrl Pts',(487.181139377683,0.,37.4129492363257));
#86612=CARTESIAN_POINT('Ctrl Pts',(487.181139377683,-37.4129492363257,37.4129492363257));
#86613=CARTESIAN_POINT('Ctrl Pts',(487.181139377683,-37.4129492363257,0.));
#86614=CARTESIAN_POINT('Ctrl Pts',(487.181139377683,-37.4129492363257,-37.4129492363257));
#86615=CARTESIAN_POINT('Ctrl Pts',(487.181139377683,0.,-37.4129492363257));
#86616=CARTESIAN_POINT('Ctrl Pts',(487.181139377683,37.4129492363257,-37.4129492363257));
#86617=CARTESIAN_POINT('Ctrl Pts',(487.181139377683,37.4129492363257,0.));
#86618=CARTESIAN_POINT('Ctrl Pts',(487.905484857346,37.4944726873275,0.));
#86619=CARTESIAN_POINT('Ctrl Pts',(487.905484857346,37.4944726873275,37.4944726873275));
#86620=CARTESIAN_POINT('Ctrl Pts',(487.905484857346,0.,37.4944726873275));
#86621=CARTESIAN_POINT('Ctrl Pts',(487.905484857346,-37.4944726873275,37.4944726873275));
#86622=CARTESIAN_POINT('Ctrl Pts',(487.905484857346,-37.4944726873275,0.));
#86623=CARTESIAN_POINT('Ctrl Pts',(487.905484857346,-37.4944726873275,-37.4944726873275));
#86624=CARTESIAN_POINT('Ctrl Pts',(487.905484857346,0.,-37.4944726873275));
#86625=CARTESIAN_POINT('Ctrl Pts',(487.905484857346,37.4944726873275,-37.4944726873275));
#86626=CARTESIAN_POINT('Ctrl Pts',(487.905484857346,37.4944726873275,0.));
#86627=CARTESIAN_POINT('Ctrl Pts',(488.591285723259,37.3658692476534,0.));
#86628=CARTESIAN_POINT('Ctrl Pts',(488.591285723259,37.3658692476534,37.3658692476534));
#86629=CARTESIAN_POINT('Ctrl Pts',(488.591285723259,0.,37.3658692476534));
#86630=CARTESIAN_POINT('Ctrl Pts',(488.591285723259,-37.3658692476534,37.3658692476534));
#86631=CARTESIAN_POINT('Ctrl Pts',(488.591285723259,-37.3658692476534,0.));
#86632=CARTESIAN_POINT('Ctrl Pts',(488.591285723259,-37.3658692476534,-37.3658692476534));
#86633=CARTESIAN_POINT('Ctrl Pts',(488.591285723259,0.,-37.3658692476534));
#86634=CARTESIAN_POINT('Ctrl Pts',(488.591285723259,37.3658692476534,-37.3658692476534));
#86635=CARTESIAN_POINT('Ctrl Pts',(488.591285723259,37.3658692476534,0.));
#86636=CARTESIAN_POINT('Ctrl Pts',(489.239790144105,36.9946079386645,0.));
#86637=CARTESIAN_POINT('Ctrl Pts',(489.239790144105,36.9946079386645,36.9946079386645));
#86638=CARTESIAN_POINT('Ctrl Pts',(489.239790144105,0.,36.9946079386645));
#86639=CARTESIAN_POINT('Ctrl Pts',(489.239790144105,-36.9946079386645,36.9946079386645));
#86640=CARTESIAN_POINT('Ctrl Pts',(489.239790144105,-36.9946079386645,0.));
#86641=CARTESIAN_POINT('Ctrl Pts',(489.239790144105,-36.9946079386645,-36.9946079386645));
#86642=CARTESIAN_POINT('Ctrl Pts',(489.239790144105,0.,-36.9946079386645));
#86643=CARTESIAN_POINT('Ctrl Pts',(489.239790144105,36.9946079386645,-36.9946079386645));
#86644=CARTESIAN_POINT('Ctrl Pts',(489.239790144105,36.9946079386645,0.));
#86645=CARTESIAN_POINT('Ctrl Pts',(489.860088758647,36.4120284644969,0.));
#86646=CARTESIAN_POINT('Ctrl Pts',(489.860088758647,36.4120284644969,36.4120284644969));
#86647=CARTESIAN_POINT('Ctrl Pts',(489.860088758647,0.,36.4120284644969));
#86648=CARTESIAN_POINT('Ctrl Pts',(489.860088758647,-36.4120284644969,36.4120284644969));
#86649=CARTESIAN_POINT('Ctrl Pts',(489.860088758647,-36.4120284644969,0.));
#86650=CARTESIAN_POINT('Ctrl Pts',(489.860088758647,-36.4120284644969,-36.4120284644969));
#86651=CARTESIAN_POINT('Ctrl Pts',(489.860088758647,0.,-36.4120284644969));
#86652=CARTESIAN_POINT('Ctrl Pts',(489.860088758647,36.4120284644969,-36.4120284644969));
#86653=CARTESIAN_POINT('Ctrl Pts',(489.860088758647,36.4120284644969,0.));
#86654=CARTESIAN_POINT('Ctrl Pts',(490.468280769547,35.7212079443224,0.));
#86655=CARTESIAN_POINT('Ctrl Pts',(490.468280769547,35.7212079443224,35.7212079443224));
#86656=CARTESIAN_POINT('Ctrl Pts',(490.468280769547,0.,35.7212079443224));
#86657=CARTESIAN_POINT('Ctrl Pts',(490.468280769547,-35.7212079443224,35.7212079443224));
#86658=CARTESIAN_POINT('Ctrl Pts',(490.468280769547,-35.7212079443224,0.));
#86659=CARTESIAN_POINT('Ctrl Pts',(490.468280769547,-35.7212079443224,-35.7212079443224));
#86660=CARTESIAN_POINT('Ctrl Pts',(490.468280769547,0.,-35.7212079443224));
#86661=CARTESIAN_POINT('Ctrl Pts',(490.468280769547,35.7212079443224,-35.7212079443224));
#86662=CARTESIAN_POINT('Ctrl Pts',(490.468280769547,35.7212079443224,0.));
#86663=CARTESIAN_POINT('Ctrl Pts',(491.082318128631,35.0575437241964,0.));
#86664=CARTESIAN_POINT('Ctrl Pts',(491.082318128631,35.0575437241964,35.0575437241964));
#86665=CARTESIAN_POINT('Ctrl Pts',(491.082318128631,0.,35.0575437241964));
#86666=CARTESIAN_POINT('Ctrl Pts',(491.082318128631,-35.0575437241964,35.0575437241964));
#86667=CARTESIAN_POINT('Ctrl Pts',(491.082318128631,-35.0575437241964,0.));
#86668=CARTESIAN_POINT('Ctrl Pts',(491.082318128631,-35.0575437241964,-35.0575437241964));
#86669=CARTESIAN_POINT('Ctrl Pts',(491.082318128631,0.,-35.0575437241964));
#86670=CARTESIAN_POINT('Ctrl Pts',(491.082318128631,35.0575437241964,-35.0575437241964));
#86671=CARTESIAN_POINT('Ctrl Pts',(491.082318128631,35.0575437241964,0.));
#86672=CARTESIAN_POINT('Ctrl Pts',(491.717567381893,34.5582390968106,0.));
#86673=CARTESIAN_POINT('Ctrl Pts',(491.717567381893,34.5582390968106,34.5582390968106));
#86674=CARTESIAN_POINT('Ctrl Pts',(491.717567381893,0.,34.5582390968106));
#86675=CARTESIAN_POINT('Ctrl Pts',(491.717567381893,-34.5582390968106,34.5582390968106));
#86676=CARTESIAN_POINT('Ctrl Pts',(491.717567381893,-34.5582390968106,0.));
#86677=CARTESIAN_POINT('Ctrl Pts',(491.717567381893,-34.5582390968106,-34.5582390968106));
#86678=CARTESIAN_POINT('Ctrl Pts',(491.717567381893,0.,-34.5582390968106));
#86679=CARTESIAN_POINT('Ctrl Pts',(491.717567381893,34.5582390968106,-34.5582390968106));
#86680=CARTESIAN_POINT('Ctrl Pts',(491.717567381893,34.5582390968106,0.));
#86681=CARTESIAN_POINT('Ctrl Pts',(492.38261638311,34.3314791673919,0.));
#86682=CARTESIAN_POINT('Ctrl Pts',(492.38261638311,34.3314791673919,34.3314791673919));
#86683=CARTESIAN_POINT('Ctrl Pts',(492.38261638311,0.,34.3314791673919));
#86684=CARTESIAN_POINT('Ctrl Pts',(492.38261638311,-34.3314791673919,34.3314791673919));
#86685=CARTESIAN_POINT('Ctrl Pts',(492.38261638311,-34.3314791673919,0.));
#86686=CARTESIAN_POINT('Ctrl Pts',(492.38261638311,-34.3314791673919,-34.3314791673919));
#86687=CARTESIAN_POINT('Ctrl Pts',(492.38261638311,0.,-34.3314791673919));
#86688=CARTESIAN_POINT('Ctrl Pts',(492.38261638311,34.3314791673919,-34.3314791673919));
#86689=CARTESIAN_POINT('Ctrl Pts',(492.38261638311,34.3314791673919,0.));
#86690=CARTESIAN_POINT('Ctrl Pts',(493.073654019524,34.4177010965138,0.));
#86691=CARTESIAN_POINT('Ctrl Pts',(493.073654019524,34.4177010965138,34.4177010965138));
#86692=CARTESIAN_POINT('Ctrl Pts',(493.073654019524,0.,34.4177010965138));
#86693=CARTESIAN_POINT('Ctrl Pts',(493.073654019524,-34.4177010965138,34.4177010965138));
#86694=CARTESIAN_POINT('Ctrl Pts',(493.073654019524,-34.4177010965138,0.));
#86695=CARTESIAN_POINT('Ctrl Pts',(493.073654019524,-34.4177010965138,-34.4177010965138));
#86696=CARTESIAN_POINT('Ctrl Pts',(493.073654019524,0.,-34.4177010965138));
#86697=CARTESIAN_POINT('Ctrl Pts',(493.073654019524,34.4177010965138,-34.4177010965138));
#86698=CARTESIAN_POINT('Ctrl Pts',(493.073654019524,34.4177010965138,0.));
#86699=CARTESIAN_POINT('Ctrl Pts',(493.775332748996,34.7899536801706,0.));
#86700=CARTESIAN_POINT('Ctrl Pts',(493.775332748996,34.7899536801706,34.7899536801706));
#86701=CARTESIAN_POINT('Ctrl Pts',(493.775332748996,0.,34.7899536801706));
#86702=CARTESIAN_POINT('Ctrl Pts',(493.775332748996,-34.7899536801706,34.7899536801706));
#86703=CARTESIAN_POINT('Ctrl Pts',(493.775332748996,-34.7899536801706,0.));
#86704=CARTESIAN_POINT('Ctrl Pts',(493.775332748996,-34.7899536801706,-34.7899536801706));
#86705=CARTESIAN_POINT('Ctrl Pts',(493.775332748996,0.,-34.7899536801706));
#86706=CARTESIAN_POINT('Ctrl Pts',(493.775332748996,34.7899536801706,-34.7899536801706));
#86707=CARTESIAN_POINT('Ctrl Pts',(493.775332748996,34.7899536801706,0.));
#86708=CARTESIAN_POINT('Ctrl Pts',(494.466408007924,35.3833258004001,0.));
#86709=CARTESIAN_POINT('Ctrl Pts',(494.466408007924,35.3833258004001,35.3833258004001));
#86710=CARTESIAN_POINT('Ctrl Pts',(494.466408007924,0.,35.3833258004001));
#86711=CARTESIAN_POINT('Ctrl Pts',(494.466408007924,-35.3833258004001,35.3833258004001));
#86712=CARTESIAN_POINT('Ctrl Pts',(494.466408007924,-35.3833258004001,0.));
#86713=CARTESIAN_POINT('Ctrl Pts',(494.466408007924,-35.3833258004001,-35.3833258004001));
#86714=CARTESIAN_POINT('Ctrl Pts',(494.466408007924,0.,-35.3833258004001));
#86715=CARTESIAN_POINT('Ctrl Pts',(494.466408007924,35.3833258004001,-35.3833258004001));
#86716=CARTESIAN_POINT('Ctrl Pts',(494.466408007924,35.3833258004001,0.));
#86717=CARTESIAN_POINT('Ctrl Pts',(495.123822940199,36.1150832766185,0.));
#86718=CARTESIAN_POINT('Ctrl Pts',(495.123822940199,36.1150832766185,36.1150832766185));
#86719=CARTESIAN_POINT('Ctrl Pts',(495.123822940199,0.,36.1150832766185));
#86720=CARTESIAN_POINT('Ctrl Pts',(495.123822940199,-36.1150832766185,36.1150832766185));
#86721=CARTESIAN_POINT('Ctrl Pts',(495.123822940199,-36.1150832766185,0.));
#86722=CARTESIAN_POINT('Ctrl Pts',(495.123822940199,-36.1150832766185,-36.1150832766185));
#86723=CARTESIAN_POINT('Ctrl Pts',(495.123822940199,0.,-36.1150832766185));
#86724=CARTESIAN_POINT('Ctrl Pts',(495.123822940199,36.1150832766185,-36.1150832766185));
#86725=CARTESIAN_POINT('Ctrl Pts',(495.123822940199,36.1150832766185,0.));
#86726=CARTESIAN_POINT('Ctrl Pts',(495.727749645427,36.9101272403245,0.));
#86727=CARTESIAN_POINT('Ctrl Pts',(495.727749645427,36.9101272403245,36.9101272403245));
#86728=CARTESIAN_POINT('Ctrl Pts',(495.727749645427,0.,36.9101272403245));
#86729=CARTESIAN_POINT('Ctrl Pts',(495.727749645427,-36.9101272403245,36.9101272403245));
#86730=CARTESIAN_POINT('Ctrl Pts',(495.727749645427,-36.9101272403245,0.));
#86731=CARTESIAN_POINT('Ctrl Pts',(495.727749645427,-36.9101272403245,-36.9101272403245));
#86732=CARTESIAN_POINT('Ctrl Pts',(495.727749645427,0.,-36.9101272403245));
#86733=CARTESIAN_POINT('Ctrl Pts',(495.727749645427,36.9101272403245,-36.9101272403245));
#86734=CARTESIAN_POINT('Ctrl Pts',(495.727749645427,36.9101272403245,0.));
#86735=CARTESIAN_POINT('Ctrl Pts',(496.265277600815,37.7196967747546,0.));
#86736=CARTESIAN_POINT('Ctrl Pts',(496.265277600815,37.7196967747546,37.7196967747546));
#86737=CARTESIAN_POINT('Ctrl Pts',(496.265277600815,0.,37.7196967747546));
#86738=CARTESIAN_POINT('Ctrl Pts',(496.265277600815,-37.7196967747546,37.7196967747546));
#86739=CARTESIAN_POINT('Ctrl Pts',(496.265277600815,-37.7196967747546,0.));
#86740=CARTESIAN_POINT('Ctrl Pts',(496.265277600815,-37.7196967747546,-37.7196967747546));
#86741=CARTESIAN_POINT('Ctrl Pts',(496.265277600815,0.,-37.7196967747546));
#86742=CARTESIAN_POINT('Ctrl Pts',(496.265277600815,37.7196967747546,-37.7196967747546));
#86743=CARTESIAN_POINT('Ctrl Pts',(496.265277600815,37.7196967747546,0.));
#86744=CARTESIAN_POINT('Ctrl Pts',(496.728598336574,38.5141264690987,0.));
#86745=CARTESIAN_POINT('Ctrl Pts',(496.728598336574,38.5141264690987,38.5141264690987));
#86746=CARTESIAN_POINT('Ctrl Pts',(496.728598336574,0.,38.5141264690987));
#86747=CARTESIAN_POINT('Ctrl Pts',(496.728598336574,-38.5141264690987,38.5141264690987));
#86748=CARTESIAN_POINT('Ctrl Pts',(496.728598336574,-38.5141264690987,0.));
#86749=CARTESIAN_POINT('Ctrl Pts',(496.728598336574,-38.5141264690987,-38.5141264690987));
#86750=CARTESIAN_POINT('Ctrl Pts',(496.728598336574,0.,-38.5141264690987));
#86751=CARTESIAN_POINT('Ctrl Pts',(496.728598336574,38.5141264690987,-38.5141264690987));
#86752=CARTESIAN_POINT('Ctrl Pts',(496.728598336574,38.5141264690987,0.));
#86753=CARTESIAN_POINT('Ctrl Pts',(497.036816221337,39.1258367553137,0.));
#86754=CARTESIAN_POINT('Ctrl Pts',(497.036816221337,39.1258367553137,39.1258367553137));
#86755=CARTESIAN_POINT('Ctrl Pts',(497.036816221337,0.,39.1258367553137));
#86756=CARTESIAN_POINT('Ctrl Pts',(497.036816221337,-39.1258367553137,39.1258367553137));
#86757=CARTESIAN_POINT('Ctrl Pts',(497.036816221337,-39.1258367553137,0.));
#86758=CARTESIAN_POINT('Ctrl Pts',(497.036816221337,-39.1258367553137,-39.1258367553137));
#86759=CARTESIAN_POINT('Ctrl Pts',(497.036816221337,0.,-39.1258367553137));
#86760=CARTESIAN_POINT('Ctrl Pts',(497.036816221337,39.1258367553137,-39.1258367553137));
#86761=CARTESIAN_POINT('Ctrl Pts',(497.036816221337,39.1258367553137,0.));
#86762=CARTESIAN_POINT('Ctrl Pts',(497.2322862177,39.5689919786325,0.));
#86763=CARTESIAN_POINT('Ctrl Pts',(497.2322862177,39.5689919786325,39.5689919786325));
#86764=CARTESIAN_POINT('Ctrl Pts',(497.2322862177,0.,39.5689919786325));
#86765=CARTESIAN_POINT('Ctrl Pts',(497.2322862177,-39.5689919786325,39.5689919786325));
#86766=CARTESIAN_POINT('Ctrl Pts',(497.2322862177,-39.5689919786325,0.));
#86767=CARTESIAN_POINT('Ctrl Pts',(497.2322862177,-39.5689919786325,-39.5689919786325));
#86768=CARTESIAN_POINT('Ctrl Pts',(497.2322862177,0.,-39.5689919786325));
#86769=CARTESIAN_POINT('Ctrl Pts',(497.2322862177,39.5689919786325,-39.5689919786325));
#86770=CARTESIAN_POINT('Ctrl Pts',(497.2322862177,39.5689919786325,0.));
#86771=CARTESIAN_POINT('Ctrl Pts',(497.346738878877,39.8574876472158,0.));
#86772=CARTESIAN_POINT('Ctrl Pts',(497.346738878877,39.8574876472158,39.8574876472158));
#86773=CARTESIAN_POINT('Ctrl Pts',(497.346738878877,0.,39.8574876472158));
#86774=CARTESIAN_POINT('Ctrl Pts',(497.346738878877,-39.8574876472158,39.8574876472158));
#86775=CARTESIAN_POINT('Ctrl Pts',(497.346738878877,-39.8574876472158,0.));
#86776=CARTESIAN_POINT('Ctrl Pts',(497.346738878877,-39.8574876472158,-39.8574876472158));
#86777=CARTESIAN_POINT('Ctrl Pts',(497.346738878877,0.,-39.8574876472158));
#86778=CARTESIAN_POINT('Ctrl Pts',(497.346738878877,39.8574876472158,-39.8574876472158));
#86779=CARTESIAN_POINT('Ctrl Pts',(497.346738878877,39.8574876472158,0.));
#86780=CARTESIAN_POINT('Ctrl Pts',(497.4,40.,0.));
#86781=CARTESIAN_POINT('Ctrl Pts',(497.4,40.,40.));
#86782=CARTESIAN_POINT('Ctrl Pts',(497.4,0.,40.));
#86783=CARTESIAN_POINT('Ctrl Pts',(497.4,-40.,40.));
#86784=CARTESIAN_POINT('Ctrl Pts',(497.4,-40.,0.));
#86785=CARTESIAN_POINT('Ctrl Pts',(497.4,-40.,-40.));
#86786=CARTESIAN_POINT('Ctrl Pts',(497.4,0.,-40.));
#86787=CARTESIAN_POINT('Ctrl Pts',(497.4,40.,-40.));
#86788=CARTESIAN_POINT('Ctrl Pts',(497.4,40.,0.));
#86789=CARTESIAN_POINT('',(431.,13.5,0.));
#86790=CARTESIAN_POINT('Ctrl Pts',(497.4,40.,0.));
#86791=CARTESIAN_POINT('Ctrl Pts',(497.346738878877,39.8574876472158,0.));
#86792=CARTESIAN_POINT('Ctrl Pts',(497.2322862177,39.5689919786325,0.));
#86793=CARTESIAN_POINT('Ctrl Pts',(497.036816221337,39.1258367553137,0.));
#86794=CARTESIAN_POINT('Ctrl Pts',(496.728598336574,38.5141264690987,0.));
#86795=CARTESIAN_POINT('Ctrl Pts',(496.265277600815,37.7196967747546,0.));
#86796=CARTESIAN_POINT('Ctrl Pts',(495.727749645427,36.9101272403245,0.));
#86797=CARTESIAN_POINT('Ctrl Pts',(495.123822940199,36.1150832766185,0.));
#86798=CARTESIAN_POINT('Ctrl Pts',(494.466408007924,35.3833258004001,0.));
#86799=CARTESIAN_POINT('Ctrl Pts',(493.775332748996,34.7899536801706,0.));
#86800=CARTESIAN_POINT('Ctrl Pts',(493.073654019524,34.4177010965138,0.));
#86801=CARTESIAN_POINT('Ctrl Pts',(492.38261638311,34.3314791673919,0.));
#86802=CARTESIAN_POINT('Ctrl Pts',(491.717567381893,34.5582390968106,0.));
#86803=CARTESIAN_POINT('Ctrl Pts',(491.082318128631,35.0575437241964,0.));
#86804=CARTESIAN_POINT('Ctrl Pts',(490.468280769547,35.7212079443224,0.));
#86805=CARTESIAN_POINT('Ctrl Pts',(489.860088758647,36.4120284644969,0.));
#86806=CARTESIAN_POINT('Ctrl Pts',(489.239790144105,36.9946079386645,0.));
#86807=CARTESIAN_POINT('Ctrl Pts',(488.591285723259,37.3658692476534,0.));
#86808=CARTESIAN_POINT('Ctrl Pts',(487.905484857346,37.4944726873275,0.));
#86809=CARTESIAN_POINT('Ctrl Pts',(487.181139377683,37.4129492363257,0.));
#86810=CARTESIAN_POINT('Ctrl Pts',(486.423221268854,37.1812508806874,0.));
#86811=CARTESIAN_POINT('Ctrl Pts',(485.641971156704,36.8618266029695,0.));
#86812=CARTESIAN_POINT('Ctrl Pts',(484.851896806652,36.4837434465982,0.));
#86813=CARTESIAN_POINT('Ctrl Pts',(484.06995894186,36.0346290589183,0.));
#86814=CARTESIAN_POINT('Ctrl Pts',(483.312607050695,35.4828759962818,0.));
#86815=CARTESIAN_POINT('Ctrl Pts',(482.593077053267,34.7923200716526,0.));
#86816=CARTESIAN_POINT('Ctrl Pts',(481.91867866565,33.939552026335,0.));
#86817=CARTESIAN_POINT('Ctrl Pts',(481.287852379122,32.9310860845041,0.));
#86818=CARTESIAN_POINT('Ctrl Pts',(480.687988617522,31.8177751379128,0.));
#86819=CARTESIAN_POINT('Ctrl Pts',(480.100216291509,30.6791487158265,0.));
#86820=CARTESIAN_POINT('Ctrl Pts',(479.503653522459,29.6103104041391,0.));
#86821=CARTESIAN_POINT('Ctrl Pts',(478.879732236756,28.7080878516033,0.));
#86822=CARTESIAN_POINT('Ctrl Pts',(478.216787070683,28.0569960770463,0.));
#86823=CARTESIAN_POINT('Ctrl Pts',(477.513843400759,27.7164651257201,0.));
#86824=CARTESIAN_POINT('Ctrl Pts',(476.786527826342,27.7044708275784,0.));
#86825=CARTESIAN_POINT('Ctrl Pts',(476.061833863912,27.999869975222,0.));
#86826=CARTESIAN_POINT('Ctrl Pts',(475.36775535895,28.5524756034697,0.));
#86827=CARTESIAN_POINT('Ctrl Pts',(474.725466937653,29.2906333134204,0.));
#86828=CARTESIAN_POINT('Ctrl Pts',(474.138366833956,30.1297846394355,0.));
#86829=CARTESIAN_POINT('Ctrl Pts',(473.589859436769,30.9807114425168,0.));
#86830=CARTESIAN_POINT('Ctrl Pts',(473.052965117723,31.7579657390958,0.));
#86831=CARTESIAN_POINT('Ctrl Pts',(472.497221742613,32.388473647408,0.));
#86832=CARTESIAN_POINT('Ctrl Pts',(471.89635548407,32.8195310910232,0.));
#86833=CARTESIAN_POINT('Ctrl Pts',(471.236383616488,33.0283632061197,0.));
#86834=CARTESIAN_POINT('Ctrl Pts',(470.521241805588,33.0271235924796,0.));
#86835=CARTESIAN_POINT('Ctrl Pts',(469.766000094273,32.8469261327295,0.));
#86836=CARTESIAN_POINT('Ctrl Pts',(468.991825973097,32.5247950832038,0.));
#86837=CARTESIAN_POINT('Ctrl Pts',(468.220253767095,32.0894344364089,0.));
#86838=CARTESIAN_POINT('Ctrl Pts',(467.467796162958,31.5476428728425,0.));
#86839=CARTESIAN_POINT('Ctrl Pts',(466.745838674916,30.8932609419353,0.));
#86840=CARTESIAN_POINT('Ctrl Pts',(466.060566868545,30.1158330796105,0.));
#86841=CARTESIAN_POINT('Ctrl Pts',(465.412818401399,29.2096983338665,0.));
#86842=CARTESIAN_POINT('Ctrl Pts',(464.798092368276,28.1821479594276,0.));
#86843=CARTESIAN_POINT('Ctrl Pts',(464.206176993335,27.0638091657224,0.));
#86844=CARTESIAN_POINT('Ctrl Pts',(463.621964437201,25.9120692248671,0.));
#86845=CARTESIAN_POINT('Ctrl Pts',(463.028833596255,24.7993805174891,0.));
#86846=CARTESIAN_POINT('Ctrl Pts',(462.411522978371,23.8046505711925,0.));
#86847=CARTESIAN_POINT('Ctrl Pts',(461.759168926054,23.0034635988083,0.));
#86848=CARTESIAN_POINT('Ctrl Pts',(461.068363394086,22.4586715684347,0.));
#86849=CARTESIAN_POINT('Ctrl Pts',(460.34599973061,22.211124033265,0.));
#86850=CARTESIAN_POINT('Ctrl Pts',(459.612787385745,22.2695103984714,0.));
#86851=CARTESIAN_POINT('Ctrl Pts',(458.89594022623,22.6137057693112,0.));
#86852=CARTESIAN_POINT('Ctrl Pts',(458.220427115088,23.1990940255842,0.));
#86853=CARTESIAN_POINT('Ctrl Pts',(457.601703267487,23.960894022917,0.));
#86854=CARTESIAN_POINT('Ctrl Pts',(457.035460070478,24.8175654564571,0.));
#86855=CARTESIAN_POINT('Ctrl Pts',(456.499992138814,25.6788942561824,0.));
#86856=CARTESIAN_POINT('Ctrl Pts',(455.965472189203,26.4565068762911,0.));
#86857=CARTESIAN_POINT('Ctrl Pts',(455.401407401473,27.0741275496278,0.));
#86858=CARTESIAN_POINT('Ctrl Pts',(454.784171241843,27.4768576432717,0.));
#86859=CARTESIAN_POINT('Ctrl Pts',(454.106137134847,27.6435191850799,0.));
#86860=CARTESIAN_POINT('Ctrl Pts',(453.378537630885,27.5886555924961,0.));
#86861=CARTESIAN_POINT('Ctrl Pts',(452.622411993808,27.3452045659704,0.));
#86862=CARTESIAN_POINT('Ctrl Pts',(451.862441449957,26.9520337795735,0.));
#86863=CARTESIAN_POINT('Ctrl Pts',(451.119142458871,26.4383182927734,0.));
#86864=CARTESIAN_POINT('Ctrl Pts',(450.403201234375,25.8128681585372,0.));
#86865=CARTESIAN_POINT('Ctrl Pts',(449.71798609425,25.074273116099,0.));
#86866=CARTESIAN_POINT('Ctrl Pts',(449.061035117611,24.2182549404179,0.));
#86867=CARTESIAN_POINT('Ctrl Pts',(448.425955791819,23.2464235854324,0.));
#86868=CARTESIAN_POINT('Ctrl Pts',(447.804096970417,22.1736869588598,0.));
#86869=CARTESIAN_POINT('Ctrl Pts',(447.186436510144,21.0380603073665,0.));
#86870=CARTESIAN_POINT('Ctrl Pts',(446.564983118453,19.9034942867493,0.));
#86871=CARTESIAN_POINT('Ctrl Pts',(445.933164114128,18.8470019997588,0.));
#86872=CARTESIAN_POINT('Ctrl Pts',(445.286408098586,17.9489859823433,0.));
#86873=CARTESIAN_POINT('Ctrl Pts',(444.622665692905,17.2822090124047,0.));
#86874=CARTESIAN_POINT('Ctrl Pts',(443.942925321305,16.9015384494366,0.));
#86875=CARTESIAN_POINT('Ctrl Pts',(443.251810955599,16.8328795404879,0.));
#86876=CARTESIAN_POINT('Ctrl Pts',(442.557926874702,17.0637870913372,0.));
#86877=CARTESIAN_POINT('Ctrl Pts',(441.871528812589,17.5520839307903,0.));
#86878=CARTESIAN_POINT('Ctrl Pts',(441.202275420219,18.2332083062446,0.));
#86879=CARTESIAN_POINT('Ctrl Pts',(440.557174885988,19.0280111167061,0.));
#86880=CARTESIAN_POINT('Ctrl Pts',(439.937886180109,19.8503961731823,0.));
#86881=CARTESIAN_POINT('Ctrl Pts',(439.341309422512,20.6146885506738,0.));
#86882=CARTESIAN_POINT('Ctrl Pts',(438.761636765821,21.2425737573923,0.));
#86883=CARTESIAN_POINT('Ctrl Pts',(438.191994671,21.6705685715134,0.));
#86884=CARTESIAN_POINT('Ctrl Pts',(437.62612331768,21.8564147928601,0.));
#86885=CARTESIAN_POINT('Ctrl Pts',(437.060372222462,21.7881221006031,0.));
#86886=CARTESIAN_POINT('Ctrl Pts',(436.493850849539,21.4807238935623,0.));
#86887=CARTESIAN_POINT('Ctrl Pts',(435.927631335713,20.9670478075204,0.));
#86888=CARTESIAN_POINT('Ctrl Pts',(435.364242124671,20.2901523149136,0.));
#86889=CARTESIAN_POINT('Ctrl Pts',(434.807068105737,19.4956986413733,0.));
#86890=CARTESIAN_POINT('Ctrl Pts',(434.260020980134,18.6299473105583,0.));
#86891=CARTESIAN_POINT('Ctrl Pts',(433.727172908933,17.7371471664815,0.));
#86892=CARTESIAN_POINT('Ctrl Pts',(433.212390321051,16.8570423033932,0.));
#86893=CARTESIAN_POINT('Ctrl Pts',(432.719002234035,16.0226042712625,0.));
#86894=CARTESIAN_POINT('Ctrl Pts',(432.249367015116,15.2569713036193,0.));
#86895=CARTESIAN_POINT('Ctrl Pts',(431.804856206642,14.5737184153466,0.));
#86896=CARTESIAN_POINT('Ctrl Pts',(431.469898541327,14.0985040583044,0.));
#86897=CARTESIAN_POINT('Ctrl Pts',(431.230394288423,13.7832480588419,0.));
#86898=CARTESIAN_POINT('Ctrl Pts',(431.075930488729,13.5913677105967,0.));
#86899=CARTESIAN_POINT('Ctrl Pts',(431.,13.5,0.));
#86900=CARTESIAN_POINT('',(431.,-13.5,-1.65327317884893E-15));
#86901=CARTESIAN_POINT('Origin',(431.,0.,0.));
#86902=CARTESIAN_POINT('Origin',(431.,0.,0.));
#86903=CARTESIAN_POINT('Origin',(430.5,0.,0.));
#86904=CARTESIAN_POINT('',(430.5,-12.75,-1.56142466891288E-15));
#90348=UNCERTAINTY_MEASURE_WITH_UNIT(LENGTH_MEASURE(0.01),#90375,
'DISTANCE_ACCURACY_VALUE',
'Maximum model space distance between geometric entities at asserted c
onnectivities');
#90355=UNCERTAINTY_MEASURE_WITH_UNIT(LENGTH_MEASURE(0.01),#90375,
'DISTANCE_ACCURACY_VALUE',
'Maximum model space distance between geometric entities at asserted c
onnectivities');
#90367=(
GEOMETRIC_REPRESENTATION_CONTEXT(3)
GLOBAL_UNCERTAINTY_ASSIGNED_CONTEXT((#90348))
GLOBAL_UNIT_ASSIGNED_CONTEXT((#90375,#90377,#90378))
REPRESENTATION_CONTEXT('','3D')
);
#90374=(
GEOMETRIC_REPRESENTATION_CONTEXT(3)
GLOBAL_UNCERTAINTY_ASSIGNED_CONTEXT((#90355))
GLOBAL_UNIT_ASSIGNED_CONTEXT((#90375,#90377,#90378))
REPRESENTATION_CONTEXT('','3D')
);
#90375=(
LENGTH_UNIT()
NAMED_UNIT(*)
SI_UNIT(.MILLI.,.METRE.)
);
#90377=(
NAMED_UNIT(*)
PLANE_ANGLE_UNIT()
SI_UNIT($,.RADIAN.)
);
#90378=(
NAMED_UNIT(*)
SI_UNIT($,.STERADIAN.)
SOLID_ANGLE_UNIT()
);
#90390=SHAPE_DEFINITION_REPRESENTATION(#90408,#90451);
#90408=PRODUCT_DEFINITION_SHAPE('',$,#90470);
#90451=SHAPE_REPRESENTATION('',(#44235),#90367);
#90458=PRODUCT_DEFINITION_CONTEXT('part definition',#90514,'design');
#90470=PRODUCT_DEFINITION('2026-10-11-12-53-12-563','11_Inner_CV_Boot',
#90488,#90458);
#90488=PRODUCT_DEFINITION_FORMATION('',$,#90527);
#90514=APPLICATION_CONTEXT(
'Core Data for Automotive Mechanical Design Process');
#90515=PRODUCT_CONTEXT('part definition',#90514,'mechanical');
#90527=PRODUCT('2026-10-11-12-53-12-563','11_Inner_CV_Boot',$,(#90515));
#90695=COLOUR_RGB('Off White',0.89,0.88,0.83);
#90696=FILL_AREA_STYLE_COLOUR('',#90695);
#90697=FILL_AREA_STYLE('',(#90696));
#90698=SURFACE_STYLE_FILL_AREA(#90697);
#90699=SURFACE_SIDE_STYLE('',(#90698));
#90700=SURFACE_STYLE_USAGE(.BOTH.,#90699);
#90701=PRESENTATION_STYLE_ASSIGNMENT((#90700));
ENDSEC;
END-ISO-10303-21;
